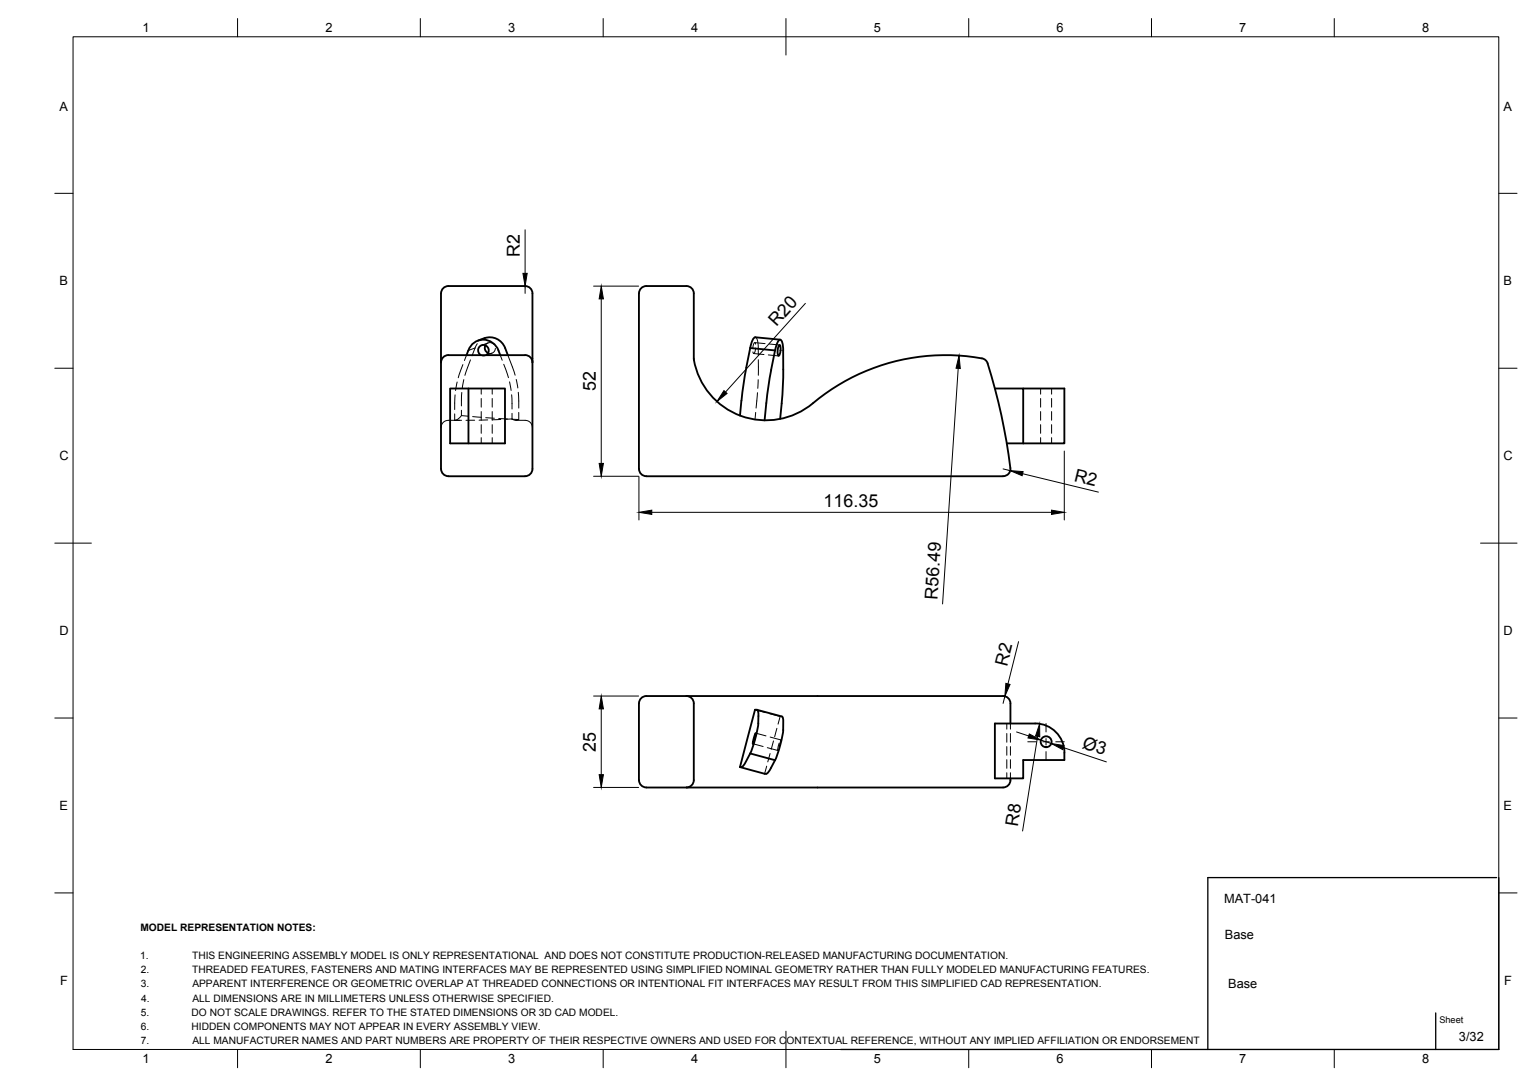
ISO-10303-21;
HEADER;
/* Generated by software containing ST-Developer
 * from STEP Tools, Inc. (www.steptools.com) 
 */

FILE_DESCRIPTION(
/* description */ ('STEP AP214'),
/* implementation_level */ '2;1');

FILE_NAME(
/* name */ 'Base.step',
/* time_stamp */ '2026-11-14T21:57:47-08:00',
/* author */ (''),
/* organization */ (''),
/* preprocessor_version */ 'ST-DEVELOPER v20.2',
/* originating_system */ 'Autodesk Translation Framework v15.17.0.0',
/* authorisation */ '');

FILE_SCHEMA (('AUTOMOTIVE_DESIGN { 1 0 10303 214 3 1 1 }'));
ENDSEC;

DATA;
#10=MECHANICAL_DESIGN_GEOMETRIC_PRESENTATION_REPRESENTATION('',(#248),#13199);
#212=SHAPE_REPRESENTATION_RELATIONSHIP('SRR','None',#13279,#230);
#230=ADVANCED_BREP_SHAPE_REPRESENTATION('',(#266),#13175);
#248=STYLED_ITEM('',(#13408),#266);
#266=MANIFOLD_SOLID_BREP('Body1',#6843);
#284=FACE_BOUND('',#2199,.T.);
#285=FACE_BOUND('',#2202,.T.);
#286=FACE_BOUND('',#2204,.T.);
#287=FACE_BOUND('',#2207,.T.);
#288=FACE_BOUND('',#2215,.T.);
#289=FACE_BOUND('',#2217,.T.);
#383=ELLIPSE('',#7086,20.7055236081625,19.9999999999245);
#384=ELLIPSE('',#7091,77.2740661068614,20.0000000018389);
#385=ELLIPSE('',#7093,20.7055236081649,19.9999999999297);
#386=ELLIPSE('',#7096,77.2740661044132,20.0000000006464);
#397=PLANE('',#7085);
#398=PLANE('',#7087);
#399=PLANE('',#7092);
#400=PLANE('',#7094);
#401=PLANE('',#7104);
#402=PLANE('',#7106);
#403=PLANE('',#7107);
#404=PLANE('',#7108);
#405=PLANE('',#7109);
#406=PLANE('',#7110);
#407=PLANE('',#7114);
#408=PLANE('',#7118);
#409=PLANE('',#7120);
#410=PLANE('',#7122);
#411=PLANE('',#7123);
#412=PLANE('',#7125);
#413=PLANE('',#7126);
#414=PLANE('',#7188);
#415=PLANE('',#7189);
#610=LINE('',#9916,#1128);
#611=LINE('',#9922,#1129);
#612=LINE('',#9928,#1130);
#613=LINE('',#9930,#1131);
#614=LINE('',#9934,#1132);
#615=LINE('',#9936,#1133);
#616=LINE('',#9938,#1134);
#617=LINE('',#9943,#1135);
#618=LINE('',#9947,#1136);
#619=LINE('',#9951,#1137);
#620=LINE('',#9957,#1138);
#621=LINE('',#9958,#1139);
#622=LINE('',#9963,#1140);
#623=LINE('',#9969,#1141);
#624=LINE('',#9975,#1142);
#625=LINE('',#9978,#1143);
#626=LINE('',#9981,#1144);
#627=LINE('',#9985,#1145);
#628=LINE('',#9990,#1146);
#629=LINE('',#9992,#1147);
#630=LINE('',#9994,#1148);
#631=LINE('',#9995,#1149);
#632=LINE('',#9997,#1150);
#633=LINE('',#10001,#1151);
#634=LINE('',#10003,#1152);
#635=LINE('',#10005,#1153);
#636=LINE('',#10006,#1154);
#637=LINE('',#10010,#1155);
#638=LINE('',#10012,#1156);
#639=LINE('',#10014,#1157);
#640=LINE('',#10015,#1158);
#641=LINE('',#10019,#1159);
#642=LINE('',#10021,#1160);
#643=LINE('',#10023,#1161);
#644=LINE('',#10024,#1162);
#645=LINE('',#10028,#1163);
#646=LINE('',#10030,#1164);
#647=LINE('',#10031,#1165);
#648=LINE('',#10032,#1166);
#649=LINE('',#10041,#1167);
#650=LINE('',#10043,#1168);
#651=LINE('',#10045,#1169);
#652=LINE('',#10046,#1170);
#653=LINE('',#10054,#1171);
#654=LINE('',#10056,#1172);
#655=LINE('',#10058,#1173);
#656=LINE('',#10059,#1174);
#657=LINE('',#10062,#1175);
#658=LINE('',#10065,#1176);
#659=LINE('',#10067,#1177);
#660=LINE('',#10068,#1178);
#661=LINE('',#10071,#1179);
#662=LINE('',#10074,#1180);
#663=LINE('',#10076,#1181);
#664=LINE('',#10077,#1182);
#665=LINE('',#10079,#1183);
#666=LINE('',#10081,#1184);
#667=LINE('',#10084,#1185);
#668=LINE('',#10147,#1186);
#669=LINE('',#10148,#1187);
#670=LINE('',#10150,#1188);
#671=LINE('',#10152,#1189);
#1128=VECTOR('',#7865,1.5);
#1129=VECTOR('',#7872,1.5);
#1130=VECTOR('',#7879,1000.);
#1131=VECTOR('',#7882,1000.);
#1132=VECTOR('',#7885,1000.);
#1133=VECTOR('',#7886,1000.);
#1134=VECTOR('',#7887,1000.);
#1135=VECTOR('',#7892,1000.);
#1136=VECTOR('',#7895,1000.);
#1137=VECTOR('',#7898,1000.);
#1138=VECTOR('',#7905,1000.);
#1139=VECTOR('',#7906,1000.);
#1140=VECTOR('',#7911,1000.);
#1141=VECTOR('',#7918,1000.);
#1142=VECTOR('',#7925,1000.);
#1143=VECTOR('',#7928,1000.);
#1144=VECTOR('',#7929,1000.);
#1145=VECTOR('',#7932,1000.);
#1146=VECTOR('',#7937,1000.);
#1147=VECTOR('',#7938,1000.);
#1148=VECTOR('',#7939,1000.);
#1149=VECTOR('',#7940,1000.);
#1150=VECTOR('',#7943,1000.);
#1151=VECTOR('',#7946,1000.);
#1152=VECTOR('',#7947,1000.);
#1153=VECTOR('',#7948,1000.);
#1154=VECTOR('',#7949,1000.);
#1155=VECTOR('',#7952,1000.);
#1156=VECTOR('',#7953,1000.);
#1157=VECTOR('',#7954,1000.);
#1158=VECTOR('',#7955,1000.);
#1159=VECTOR('',#7958,1000.);
#1160=VECTOR('',#7959,1000.);
#1161=VECTOR('',#7960,1000.);
#1162=VECTOR('',#7961,1000.);
#1163=VECTOR('',#7964,1000.);
#1164=VECTOR('',#7965,1000.);
#1165=VECTOR('',#7966,1000.);
#1166=VECTOR('',#7967,1000.);
#1167=VECTOR('',#7976,1000.);
#1168=VECTOR('',#7977,1000.);
#1169=VECTOR('',#7978,1000.);
#1170=VECTOR('',#7979,1000.);
#1171=VECTOR('',#7988,1000.);
#1172=VECTOR('',#7989,1000.);
#1173=VECTOR('',#7990,1000.);
#1174=VECTOR('',#7991,1000.);
#1175=VECTOR('',#7994,1000.);
#1176=VECTOR('',#7997,1000.);
#1177=VECTOR('',#7998,1000.);
#1178=VECTOR('',#7999,1000.);
#1179=VECTOR('',#8002,1000.);
#1180=VECTOR('',#8005,1000.);
#1181=VECTOR('',#8006,1000.);
#1182=VECTOR('',#8007,1000.);
#1183=VECTOR('',#8010,1000.);
#1184=VECTOR('',#8013,1000.);
#1185=VECTOR('',#8018,1000.);
#1186=VECTOR('',#8143,1000.);
#1187=VECTOR('',#8144,1000.);
#1188=VECTOR('',#8147,1000.);
#1189=VECTOR('',#8150,1000.);
#1646=CYLINDRICAL_SURFACE('',#7076,1.5);
#1647=CYLINDRICAL_SURFACE('',#7079,1.5);
#1648=CYLINDRICAL_SURFACE('',#7082,56.4897440054506);
#1649=CYLINDRICAL_SURFACE('',#7099,163.25688730188);
#1650=CYLINDRICAL_SURFACE('',#7105,20.);
#1651=CYLINDRICAL_SURFACE('',#7124,8.);
#1652=CYLINDRICAL_SURFACE('',#7127,2.);
#1653=CYLINDRICAL_SURFACE('',#7136,2.);
#1654=CYLINDRICAL_SURFACE('',#7138,2.);
#1655=CYLINDRICAL_SURFACE('',#7140,2.);
#1656=CYLINDRICAL_SURFACE('',#7141,2.);
#1657=CYLINDRICAL_SURFACE('',#7143,2.);
#1658=CYLINDRICAL_SURFACE('',#7153,2.);
#1659=CYLINDRICAL_SURFACE('',#7155,2.);
#1660=CYLINDRICAL_SURFACE('',#7157,2.);
#1661=CYLINDRICAL_SURFACE('',#7163,2.);
#1662=CYLINDRICAL_SURFACE('',#7165,2.);
#1663=CYLINDRICAL_SURFACE('',#7175,2.);
#1664=CYLINDRICAL_SURFACE('',#7177,2.);
#1665=CYLINDRICAL_SURFACE('',#7179,2.);
#1666=CYLINDRICAL_SURFACE('',#7187,4.54881469766181);
#1667=CYLINDRICAL_SURFACE('',#7190,25.);
#1668=CYLINDRICAL_SURFACE('',#7191,25.);
#1789=SPHERICAL_SURFACE('',#7072,2.);
#1790=SPHERICAL_SURFACE('',#7130,2.);
#1791=SPHERICAL_SURFACE('',#7133,2.);
#1792=SPHERICAL_SURFACE('',#7146,2.);
#1793=SPHERICAL_SURFACE('',#7148,2.);
#1794=SPHERICAL_SURFACE('',#7151,2.);
#1795=SPHERICAL_SURFACE('',#7167,2.);
#1796=SPHERICAL_SURFACE('',#7171,2.);
#1797=SPHERICAL_SURFACE('',#7173,2.);
#1798=SPHERICAL_SURFACE('',#7184,2.);
#1800=FACE_OUTER_BOUND('',#2191,.T.);
#1801=FACE_OUTER_BOUND('',#2192,.T.);
#1802=FACE_OUTER_BOUND('',#2193,.T.);
#1803=FACE_OUTER_BOUND('',#2194,.T.);
#1804=FACE_OUTER_BOUND('',#2195,.T.);
#1805=FACE_OUTER_BOUND('',#2196,.T.);
#1806=FACE_OUTER_BOUND('',#2197,.T.);
#1807=FACE_OUTER_BOUND('',#2198,.T.);
#1808=FACE_OUTER_BOUND('',#2200,.T.);
#1809=FACE_OUTER_BOUND('',#2201,.T.);
#1810=FACE_OUTER_BOUND('',#2203,.T.);
#1811=FACE_OUTER_BOUND('',#2205,.T.);
#1812=FACE_OUTER_BOUND('',#2206,.T.);
#1813=FACE_OUTER_BOUND('',#2208,.T.);
#1814=FACE_OUTER_BOUND('',#2209,.T.);
#1815=FACE_OUTER_BOUND('',#2210,.T.);
#1816=FACE_OUTER_BOUND('',#2211,.T.);
#1817=FACE_OUTER_BOUND('',#2212,.T.);
#1818=FACE_OUTER_BOUND('',#2213,.T.);
#1819=FACE_OUTER_BOUND('',#2214,.T.);
#1820=FACE_OUTER_BOUND('',#2216,.T.);
#1821=FACE_OUTER_BOUND('',#2218,.T.);
#1822=FACE_OUTER_BOUND('',#2219,.T.);
#1823=FACE_OUTER_BOUND('',#2220,.T.);
#1824=FACE_OUTER_BOUND('',#2221,.T.);
#1825=FACE_OUTER_BOUND('',#2222,.T.);
#1826=FACE_OUTER_BOUND('',#2223,.T.);
#1827=FACE_OUTER_BOUND('',#2224,.T.);
#1828=FACE_OUTER_BOUND('',#2225,.T.);
#1829=FACE_OUTER_BOUND('',#2226,.T.);
#1830=FACE_OUTER_BOUND('',#2227,.T.);
#1831=FACE_OUTER_BOUND('',#2228,.T.);
#1832=FACE_OUTER_BOUND('',#2229,.T.);
#1833=FACE_OUTER_BOUND('',#2230,.T.);
#1834=FACE_OUTER_BOUND('',#2231,.T.);
#1835=FACE_OUTER_BOUND('',#2232,.T.);
#1836=FACE_OUTER_BOUND('',#2233,.T.);
#1837=FACE_OUTER_BOUND('',#2234,.T.);
#1838=FACE_OUTER_BOUND('',#2235,.T.);
#1839=FACE_OUTER_BOUND('',#2236,.T.);
#1840=FACE_OUTER_BOUND('',#2237,.T.);
#1841=FACE_OUTER_BOUND('',#2238,.T.);
#1842=FACE_OUTER_BOUND('',#2239,.T.);
#1843=FACE_OUTER_BOUND('',#2240,.T.);
#1844=FACE_OUTER_BOUND('',#2241,.T.);
#1845=FACE_OUTER_BOUND('',#2242,.T.);
#1846=FACE_OUTER_BOUND('',#2243,.T.);
#1847=FACE_OUTER_BOUND('',#2244,.T.);
#1848=FACE_OUTER_BOUND('',#2245,.T.);
#1849=FACE_OUTER_BOUND('',#2246,.T.);
#1850=FACE_OUTER_BOUND('',#2247,.T.);
#1851=FACE_OUTER_BOUND('',#2248,.T.);
#1852=FACE_OUTER_BOUND('',#2249,.T.);
#1853=FACE_OUTER_BOUND('',#2250,.T.);
#1854=FACE_OUTER_BOUND('',#2251,.T.);
#1855=FACE_OUTER_BOUND('',#2252,.T.);
#1856=FACE_OUTER_BOUND('',#2253,.T.);
#1857=FACE_OUTER_BOUND('',#2254,.T.);
#1858=FACE_OUTER_BOUND('',#2255,.T.);
#1859=FACE_OUTER_BOUND('',#2256,.T.);
#2191=EDGE_LOOP('',(#4558,#4559,#4560,#4561));
#2192=EDGE_LOOP('',(#4562,#4563,#4564,#4565));
#2193=EDGE_LOOP('',(#4566,#4567,#4568));
#2194=EDGE_LOOP('',(#4569,#4570,#4571,#4572));
#2195=EDGE_LOOP('',(#4573,#4574,#4575,#4576));
#2196=EDGE_LOOP('',(#4577,#4578,#4579,#4580));
#2197=EDGE_LOOP('',(#4581,#4582,#4583,#4584));
#2198=EDGE_LOOP('',(#4585,#4586,#4587,#4588,#4589,#4590,#4591,#4592));
#2199=EDGE_LOOP('',(#4593));
#2200=EDGE_LOOP('',(#4594,#4595,#4596,#4597));
#2201=EDGE_LOOP('',(#4598,#4599,#4600,#4601,#4602,#4603,#4604,#4605));
#2202=EDGE_LOOP('',(#4606));
#2203=EDGE_LOOP('',(#4607,#4608,#4609,#4610));
#2204=EDGE_LOOP('',(#4611,#4612,#4613,#4614));
#2205=EDGE_LOOP('',(#4615,#4616,#4617,#4618));
#2206=EDGE_LOOP('',(#4619,#4620,#4621,#4622));
#2207=EDGE_LOOP('',(#4623,#4624,#4625,#4626));
#2208=EDGE_LOOP('',(#4627,#4628,#4629,#4630));
#2209=EDGE_LOOP('',(#4631,#4632,#4633,#4634));
#2210=EDGE_LOOP('',(#4635,#4636,#4637,#4638));
#2211=EDGE_LOOP('',(#4639,#4640,#4641,#4642));
#2212=EDGE_LOOP('',(#4643,#4644,#4645,#4646,#4647,#4648,#4649,#4650));
#2213=EDGE_LOOP('',(#4651,#4652,#4653,#4654,#4655,#4656,#4657,#4658));
#2214=EDGE_LOOP('',(#4659,#4660,#4661,#4662,#4663,#4664,#4665));
#2215=EDGE_LOOP('',(#4666));
#2216=EDGE_LOOP('',(#4667,#4668,#4669,#4670,#4671,#4672,#4673));
#2217=EDGE_LOOP('',(#4674));
#2218=EDGE_LOOP('',(#4675,#4676,#4677,#4678));
#2219=EDGE_LOOP('',(#4679,#4680,#4681,#4682));
#2220=EDGE_LOOP('',(#4683,#4684,#4685,#4686));
#2221=EDGE_LOOP('',(#4687,#4688,#4689,#4690));
#2222=EDGE_LOOP('',(#4691,#4692,#4693,#4694));
#2223=EDGE_LOOP('',(#4695,#4696,#4697,#4698));
#2224=EDGE_LOOP('',(#4699,#4700,#4701));
#2225=EDGE_LOOP('',(#4702,#4703,#4704));
#2226=EDGE_LOOP('',(#4705,#4706,#4707,#4708));
#2227=EDGE_LOOP('',(#4709,#4710,#4711,#4712));
#2228=EDGE_LOOP('',(#4713,#4714,#4715,#4716));
#2229=EDGE_LOOP('',(#4717,#4718,#4719,#4720));
#2230=EDGE_LOOP('',(#4721,#4722,#4723,#4724));
#2231=EDGE_LOOP('',(#4725,#4726,#4727));
#2232=EDGE_LOOP('',(#4728,#4729,#4730));
#2233=EDGE_LOOP('',(#4731,#4732,#4733));
#2234=EDGE_LOOP('',(#4734,#4735,#4736,#4737));
#2235=EDGE_LOOP('',(#4738,#4739,#4740,#4741));
#2236=EDGE_LOOP('',(#4742,#4743,#4744,#4745));
#2237=EDGE_LOOP('',(#4746,#4747,#4748,#4749));
#2238=EDGE_LOOP('',(#4750,#4751,#4752,#4753));
#2239=EDGE_LOOP('',(#4754,#4755,#4756,#4757));
#2240=EDGE_LOOP('',(#4758,#4759,#4760,#4761));
#2241=EDGE_LOOP('',(#4762,#4763,#4764));
#2242=EDGE_LOOP('',(#4765,#4766,#4767,#4768));
#2243=EDGE_LOOP('',(#4769,#4770,#4771));
#2244=EDGE_LOOP('',(#4772,#4773,#4774));
#2245=EDGE_LOOP('',(#4775,#4776,#4777,#4778));
#2246=EDGE_LOOP('',(#4779,#4780,#4781,#4782));
#2247=EDGE_LOOP('',(#4783,#4784,#4785,#4786));
#2248=EDGE_LOOP('',(#4787,#4788,#4789,#4790));
#2249=EDGE_LOOP('',(#4791,#4792,#4793,#4794));
#2250=EDGE_LOOP('',(#4795,#4796,#4797));
#2251=EDGE_LOOP('',(#4798,#4799,#4800,#4801));
#2252=EDGE_LOOP('',(#4802,#4803,#4804,#4805));
#2253=EDGE_LOOP('',(#4806,#4807,#4808,#4809));
#2254=EDGE_LOOP('',(#4810,#4811,#4812,#4813));
#2255=EDGE_LOOP('',(#4814,#4815,#4816,#4817));
#2256=EDGE_LOOP('',(#4818,#4819,#4820,#4821));
#2681=CIRCLE('',#7063,22.);
#2682=CIRCLE('',#7064,2.);
#2683=CIRCLE('',#7065,20.);
#2684=CIRCLE('',#7066,2.);
#2685=CIRCLE('',#7068,20.);
#2686=CIRCLE('',#7069,2.);
#2687=CIRCLE('',#7070,22.);
#2688=CIRCLE('',#7071,2.);
#2689=CIRCLE('',#7073,2.);
#2690=CIRCLE('',#7074,2.);
#2691=CIRCLE('',#7075,2.);
#2692=CIRCLE('',#7077,1.5);
#2693=CIRCLE('',#7078,1.5);
#2694=CIRCLE('',#7080,1.5);
#2695=CIRCLE('',#7081,1.5);
#2696=CIRCLE('',#7083,56.4897440054506);
#2697=CIRCLE('',#7084,56.4897440054506);
#2698=CIRCLE('',#7088,25.);
#2699=CIRCLE('',#7089,4.54881469766181);
#2700=CIRCLE('',#7090,25.);
#2701=CIRCLE('',#7095,25.);
#2702=CIRCLE('',#7097,25.);
#2703=CIRCLE('',#7098,4.54881469766181);
#2704=CIRCLE('',#7100,163.25688730188);
#2705=CIRCLE('',#7101,163.25688730188);
#2706=CIRCLE('',#7102,163.25688730188);
#2707=CIRCLE('',#7103,163.25688730188);
#2708=CIRCLE('',#7111,161.25688730188);
#2709=CIRCLE('',#7112,54.4897440054506);
#2710=CIRCLE('',#7113,4.);
#2711=CIRCLE('',#7115,4.);
#2712=CIRCLE('',#7116,54.4897440054506);
#2713=CIRCLE('',#7117,161.25688730188);
#2714=CIRCLE('',#7119,8.);
#2715=CIRCLE('',#7121,8.00000000000001);
#2716=CIRCLE('',#7128,2.);
#2717=CIRCLE('',#7129,2.);
#2718=CIRCLE('',#7131,2.);
#2719=CIRCLE('',#7132,2.);
#2720=CIRCLE('',#7134,2.);
#2721=CIRCLE('',#7135,2.);
#2722=CIRCLE('',#7137,2.);
#2723=CIRCLE('',#7139,2.);
#2724=CIRCLE('',#7142,2.);
#2725=CIRCLE('',#7144,2.);
#2726=CIRCLE('',#7145,2.);
#2727=CIRCLE('',#7147,2.);
#2728=CIRCLE('',#7149,2.);
#2729=CIRCLE('',#7150,2.);
#2730=CIRCLE('',#7152,2.);
#2731=CIRCLE('',#7154,2.);
#2732=CIRCLE('',#7156,2.);
#2733=CIRCLE('',#7158,2.);
#2734=CIRCLE('',#7160,2.);
#2735=CIRCLE('',#7162,2.00000000000001);
#2736=CIRCLE('',#7164,2.);
#2737=CIRCLE('',#7166,2.);
#2738=CIRCLE('',#7168,2.);
#2739=CIRCLE('',#7170,2.);
#2740=CIRCLE('',#7172,2.);
#2741=CIRCLE('',#7174,2.);
#2742=CIRCLE('',#7176,2.);
#2743=CIRCLE('',#7178,2.);
#2744=CIRCLE('',#7180,2.);
#2745=CIRCLE('',#7182,2.);
#2746=CIRCLE('',#7185,2.);
#3000=VERTEX_POINT('',#9888);
#3001=VERTEX_POINT('',#9889);
#3002=VERTEX_POINT('',#9891);
#3003=VERTEX_POINT('',#9893);
#3004=VERTEX_POINT('',#9897);
#3005=VERTEX_POINT('',#9898);
#3006=VERTEX_POINT('',#9900);
#3007=VERTEX_POINT('',#9902);
#3008=VERTEX_POINT('',#9906);
#3009=VERTEX_POINT('',#9907);
#3010=VERTEX_POINT('',#9909);
#3011=VERTEX_POINT('',#9913);
#3012=VERTEX_POINT('',#9915);
#3013=VERTEX_POINT('',#9919);
#3014=VERTEX_POINT('',#9921);
#3015=VERTEX_POINT('',#9925);
#3016=VERTEX_POINT('',#9927);
#3017=VERTEX_POINT('',#9932);
#3018=VERTEX_POINT('',#9933);
#3019=VERTEX_POINT('',#9935);
#3020=VERTEX_POINT('',#9937);
#3021=VERTEX_POINT('',#9941);
#3022=VERTEX_POINT('',#9942);
#3023=VERTEX_POINT('',#9944);
#3024=VERTEX_POINT('',#9946);
#3025=VERTEX_POINT('',#9948);
#3026=VERTEX_POINT('',#9950);
#3027=VERTEX_POINT('',#9955);
#3028=VERTEX_POINT('',#9956);
#3029=VERTEX_POINT('',#9961);
#3030=VERTEX_POINT('',#9962);
#3031=VERTEX_POINT('',#9966);
#3032=VERTEX_POINT('',#9968);
#3033=VERTEX_POINT('',#9972);
#3034=VERTEX_POINT('',#9973);
#3035=VERTEX_POINT('',#9976);
#3036=VERTEX_POINT('',#9979);
#3037=VERTEX_POINT('',#9980);
#3038=VERTEX_POINT('',#9982);
#3039=VERTEX_POINT('',#9984);
#3040=VERTEX_POINT('',#9988);
#3041=VERTEX_POINT('',#9989);
#3042=VERTEX_POINT('',#9991);
#3043=VERTEX_POINT('',#9993);
#3044=VERTEX_POINT('',#9999);
#3045=VERTEX_POINT('',#10000);
#3046=VERTEX_POINT('',#10002);
#3047=VERTEX_POINT('',#10004);
#3048=VERTEX_POINT('',#10008);
#3049=VERTEX_POINT('',#10009);
#3050=VERTEX_POINT('',#10011);
#3051=VERTEX_POINT('',#10013);
#3052=VERTEX_POINT('',#10017);
#3053=VERTEX_POINT('',#10018);
#3054=VERTEX_POINT('',#10020);
#3055=VERTEX_POINT('',#10022);
#3056=VERTEX_POINT('',#10026);
#3057=VERTEX_POINT('',#10027);
#3058=VERTEX_POINT('',#10029);
#3059=VERTEX_POINT('',#10034);
#3060=VERTEX_POINT('',#10035);
#3061=VERTEX_POINT('',#10038);
#3062=VERTEX_POINT('',#10040);
#3063=VERTEX_POINT('',#10042);
#3064=VERTEX_POINT('',#10044);
#3065=VERTEX_POINT('',#10048);
#3066=VERTEX_POINT('',#10050);
#3067=VERTEX_POINT('',#10053);
#3068=VERTEX_POINT('',#10055);
#3069=VERTEX_POINT('',#10057);
#3070=VERTEX_POINT('',#10061);
#3071=VERTEX_POINT('',#10063);
#3072=VERTEX_POINT('',#10066);
#3073=VERTEX_POINT('',#10070);
#3074=VERTEX_POINT('',#10072);
#3075=VERTEX_POINT('',#10075);
#3616=EDGE_CURVE('',#3000,#3001,#2681,.T.);
#3617=EDGE_CURVE('',#3002,#3000,#2682,.T.);
#3618=EDGE_CURVE('',#3003,#3002,#2683,.T.);
#3619=EDGE_CURVE('',#3003,#3001,#2684,.T.);
#3620=EDGE_CURVE('',#3004,#3005,#2685,.T.);
#3621=EDGE_CURVE('',#3006,#3004,#2686,.T.);
#3622=EDGE_CURVE('',#3007,#3006,#2687,.T.);
#3623=EDGE_CURVE('',#3005,#3007,#2688,.T.);
#3624=EDGE_CURVE('',#3008,#3009,#2689,.T.);
#3625=EDGE_CURVE('',#3008,#3010,#2690,.T.);
#3626=EDGE_CURVE('',#3009,#3010,#2691,.T.);
#3627=EDGE_CURVE('',#3011,#3011,#2692,.T.);
#3628=EDGE_CURVE('',#3011,#3012,#610,.T.);
#3629=EDGE_CURVE('',#3012,#3012,#2693,.T.);
#3630=EDGE_CURVE('',#3013,#3013,#2694,.T.);
#3631=EDGE_CURVE('',#3013,#3014,#611,.T.);
#3632=EDGE_CURVE('',#3014,#3014,#2695,.T.);
#3633=EDGE_CURVE('',#3002,#3015,#2696,.T.);
#3634=EDGE_CURVE('',#3015,#3016,#612,.T.);
#3635=EDGE_CURVE('',#3016,#3004,#2697,.T.);
#3636=EDGE_CURVE('',#3002,#3004,#613,.T.);
#3637=EDGE_CURVE('',#3017,#3018,#614,.T.);
#3638=EDGE_CURVE('',#3017,#3019,#615,.T.);
#3639=EDGE_CURVE('',#3019,#3020,#616,.T.);
#3640=EDGE_CURVE('',#3018,#3020,#383,.T.);
#3641=EDGE_CURVE('',#3021,#3022,#617,.T.);
#3642=EDGE_CURVE('',#3021,#3023,#2698,.T.);
#3643=EDGE_CURVE('',#3023,#3024,#618,.T.);
#3644=EDGE_CURVE('',#3024,#3025,#2699,.T.);
#3645=EDGE_CURVE('',#3025,#3026,#619,.T.);
#3646=EDGE_CURVE('',#3026,#3017,#2700,.T.);
#3647=EDGE_CURVE('',#3022,#3018,#384,.T.);
#3648=EDGE_CURVE('',#3027,#3028,#620,.T.);
#3649=EDGE_CURVE('',#3027,#3021,#621,.T.);
#3650=EDGE_CURVE('',#3028,#3022,#385,.T.);
#3651=EDGE_CURVE('',#3029,#3030,#622,.T.);
#3652=EDGE_CURVE('',#3029,#3027,#2701,.T.);
#3653=EDGE_CURVE('',#3020,#3028,#386,.T.);
#3654=EDGE_CURVE('',#3019,#3031,#2702,.T.);
#3655=EDGE_CURVE('',#3032,#3031,#623,.T.);
#3656=EDGE_CURVE('',#3030,#3032,#2703,.T.);
#3657=EDGE_CURVE('',#3033,#3034,#2704,.T.);
#3658=EDGE_CURVE('',#3034,#3009,#624,.T.);
#3659=EDGE_CURVE('',#3009,#3035,#2705,.T.);
#3660=EDGE_CURVE('',#3035,#3033,#625,.T.);
#3661=EDGE_CURVE('',#3036,#3037,#626,.T.);
#3662=EDGE_CURVE('',#3038,#3037,#2706,.T.);
#3663=EDGE_CURVE('',#3039,#3038,#627,.T.);
#3664=EDGE_CURVE('',#3036,#3039,#2707,.T.);
#3665=EDGE_CURVE('',#3040,#3041,#628,.T.);
#3666=EDGE_CURVE('',#3042,#3040,#629,.T.);
#3667=EDGE_CURVE('',#3042,#3043,#630,.T.);
#3668=EDGE_CURVE('',#3041,#3043,#631,.T.);
#3669=EDGE_CURVE('',#3005,#3003,#632,.T.);
#3670=EDGE_CURVE('',#3044,#3045,#633,.T.);
#3671=EDGE_CURVE('',#3045,#3046,#634,.T.);
#3672=EDGE_CURVE('',#3046,#3047,#635,.T.);
#3673=EDGE_CURVE('',#3047,#3044,#636,.T.);
#3674=EDGE_CURVE('',#3048,#3049,#637,.T.);
#3675=EDGE_CURVE('',#3049,#3050,#638,.T.);
#3676=EDGE_CURVE('',#3050,#3051,#639,.T.);
#3677=EDGE_CURVE('',#3051,#3048,#640,.T.);
#3678=EDGE_CURVE('',#3052,#3053,#641,.T.);
#3679=EDGE_CURVE('',#3053,#3054,#642,.T.);
#3680=EDGE_CURVE('',#3054,#3055,#643,.T.);
#3681=EDGE_CURVE('',#3055,#3052,#644,.T.);
#3682=EDGE_CURVE('',#3056,#3057,#645,.T.);
#3683=EDGE_CURVE('',#3057,#3058,#646,.T.);
#3684=EDGE_CURVE('',#3058,#3008,#647,.T.);
#3685=EDGE_CURVE('',#3008,#3056,#648,.T.);
#3686=EDGE_CURVE('',#3059,#3060,#2708,.T.);
#3687=EDGE_CURVE('',#3060,#3000,#2709,.T.);
#3688=EDGE_CURVE('',#3061,#3001,#2710,.T.);
#3689=EDGE_CURVE('',#3061,#3062,#649,.T.);
#3690=EDGE_CURVE('',#3062,#3063,#650,.T.);
#3691=EDGE_CURVE('',#3063,#3064,#651,.T.);
#3692=EDGE_CURVE('',#3064,#3059,#652,.T.);
#3693=EDGE_CURVE('',#3007,#3065,#2711,.T.);
#3694=EDGE_CURVE('',#3006,#3066,#2712,.T.);
#3695=EDGE_CURVE('',#3066,#3010,#2713,.T.);
#3696=EDGE_CURVE('',#3010,#3067,#653,.T.);
#3697=EDGE_CURVE('',#3067,#3068,#654,.T.);
#3698=EDGE_CURVE('',#3068,#3069,#655,.T.);
#3699=EDGE_CURVE('',#3069,#3065,#656,.T.);
#3700=EDGE_CURVE('',#3036,#3070,#657,.T.);
#3701=EDGE_CURVE('',#3070,#3071,#2714,.T.);
#3702=EDGE_CURVE('',#3071,#3043,#658,.T.);
#3703=EDGE_CURVE('',#3072,#3042,#659,.T.);
#3704=EDGE_CURVE('',#3037,#3072,#660,.T.);
#3705=EDGE_CURVE('',#3073,#3041,#661,.T.);
#3706=EDGE_CURVE('',#3073,#3074,#2715,.T.);
#3707=EDGE_CURVE('',#3039,#3074,#662,.T.);
#3708=EDGE_CURVE('',#3075,#3038,#663,.T.);
#3709=EDGE_CURVE('',#3075,#3040,#664,.T.);
#3710=EDGE_CURVE('',#3071,#3073,#665,.T.);
#3711=EDGE_CURVE('',#3074,#3070,#666,.T.);
#3712=EDGE_CURVE('',#3072,#3075,#667,.T.);
#3713=EDGE_CURVE('',#3068,#3054,#2716,.T.);
#3714=EDGE_CURVE('',#3055,#3067,#2717,.T.);
#3715=EDGE_CURVE('',#3068,#3051,#2718,.T.);
#3716=EDGE_CURVE('',#3051,#3054,#2719,.T.);
#3717=EDGE_CURVE('',#3055,#3058,#2720,.T.);
#3718=EDGE_CURVE('',#3058,#3067,#2721,.T.);
#3719=EDGE_CURVE('',#3048,#3053,#2722,.T.);
#3720=EDGE_CURVE('',#3069,#3050,#2723,.T.);
#3721=EDGE_CURVE('',#3052,#3057,#2724,.T.);
#3722=EDGE_CURVE('',#3053,#3063,#2725,.T.);
#3723=EDGE_CURVE('',#3064,#3052,#2726,.T.);
#3724=EDGE_CURVE('',#3048,#3063,#2727,.T.);
#3725=EDGE_CURVE('',#3069,#3047,#2728,.T.);
#3726=EDGE_CURVE('',#3047,#3050,#2729,.T.);
#3727=EDGE_CURVE('',#3064,#3057,#2730,.T.);
#3728=EDGE_CURVE('',#3049,#3062,#2731,.T.);
#3729=EDGE_CURVE('',#3044,#3049,#2732,.T.);
#3730=EDGE_CURVE('',#3065,#3046,#2733,.T.);
#3731=EDGE_CURVE('',#3066,#3016,#2734,.T.);
#3732=EDGE_CURVE('',#3035,#3066,#2735,.T.);
#3733=EDGE_CURVE('',#3056,#3034,#2736,.T.);
#3734=EDGE_CURVE('',#3059,#3056,#2737,.T.);
#3735=EDGE_CURVE('',#3044,#3062,#2738,.T.);
#3736=EDGE_CURVE('',#3005,#3046,#2739,.T.);
#3737=EDGE_CURVE('',#3035,#3016,#2740,.T.);
#3738=EDGE_CURVE('',#3059,#3034,#2741,.T.);
#3739=EDGE_CURVE('',#3045,#3061,#2742,.T.);
#3740=EDGE_CURVE('',#3003,#3045,#2743,.T.);
#3741=EDGE_CURVE('',#3033,#3015,#2744,.T.);
#3742=EDGE_CURVE('',#3060,#3033,#2745,.T.);
#3743=EDGE_CURVE('',#3060,#3015,#2746,.T.);
#3744=EDGE_CURVE('',#3032,#3025,#668,.T.);
#3745=EDGE_CURVE('',#3030,#3024,#669,.T.);
#3746=EDGE_CURVE('',#3031,#3026,#670,.T.);
#3747=EDGE_CURVE('',#3023,#3029,#671,.T.);
#4558=ORIENTED_EDGE('',*,*,#3616,.F.);
#4559=ORIENTED_EDGE('',*,*,#3617,.F.);
#4560=ORIENTED_EDGE('',*,*,#3618,.F.);
#4561=ORIENTED_EDGE('',*,*,#3619,.T.);
#4562=ORIENTED_EDGE('',*,*,#3620,.F.);
#4563=ORIENTED_EDGE('',*,*,#3621,.F.);
#4564=ORIENTED_EDGE('',*,*,#3622,.F.);
#4565=ORIENTED_EDGE('',*,*,#3623,.F.);
#4566=ORIENTED_EDGE('',*,*,#3624,.F.);
#4567=ORIENTED_EDGE('',*,*,#3625,.T.);
#4568=ORIENTED_EDGE('',*,*,#3626,.F.);
#4569=ORIENTED_EDGE('',*,*,#3627,.T.);
#4570=ORIENTED_EDGE('',*,*,#3628,.T.);
#4571=ORIENTED_EDGE('',*,*,#3629,.T.);
#4572=ORIENTED_EDGE('',*,*,#3628,.F.);
#4573=ORIENTED_EDGE('',*,*,#3630,.T.);
#4574=ORIENTED_EDGE('',*,*,#3631,.T.);
#4575=ORIENTED_EDGE('',*,*,#3632,.T.);
#4576=ORIENTED_EDGE('',*,*,#3631,.F.);
#4577=ORIENTED_EDGE('',*,*,#3633,.T.);
#4578=ORIENTED_EDGE('',*,*,#3634,.T.);
#4579=ORIENTED_EDGE('',*,*,#3635,.T.);
#4580=ORIENTED_EDGE('',*,*,#3636,.F.);
#4581=ORIENTED_EDGE('',*,*,#3637,.F.);
#4582=ORIENTED_EDGE('',*,*,#3638,.T.);
#4583=ORIENTED_EDGE('',*,*,#3639,.T.);
#4584=ORIENTED_EDGE('',*,*,#3640,.F.);
#4585=ORIENTED_EDGE('',*,*,#3641,.F.);
#4586=ORIENTED_EDGE('',*,*,#3642,.T.);
#4587=ORIENTED_EDGE('',*,*,#3643,.T.);
#4588=ORIENTED_EDGE('',*,*,#3644,.T.);
#4589=ORIENTED_EDGE('',*,*,#3645,.T.);
#4590=ORIENTED_EDGE('',*,*,#3646,.T.);
#4591=ORIENTED_EDGE('',*,*,#3637,.T.);
#4592=ORIENTED_EDGE('',*,*,#3647,.F.);
#4593=ORIENTED_EDGE('',*,*,#3629,.F.);
#4594=ORIENTED_EDGE('',*,*,#3648,.F.);
#4595=ORIENTED_EDGE('',*,*,#3649,.T.);
#4596=ORIENTED_EDGE('',*,*,#3641,.T.);
#4597=ORIENTED_EDGE('',*,*,#3650,.F.);
#4598=ORIENTED_EDGE('',*,*,#3651,.F.);
#4599=ORIENTED_EDGE('',*,*,#3652,.T.);
#4600=ORIENTED_EDGE('',*,*,#3648,.T.);
#4601=ORIENTED_EDGE('',*,*,#3653,.F.);
#4602=ORIENTED_EDGE('',*,*,#3639,.F.);
#4603=ORIENTED_EDGE('',*,*,#3654,.T.);
#4604=ORIENTED_EDGE('',*,*,#3655,.F.);
#4605=ORIENTED_EDGE('',*,*,#3656,.F.);
#4606=ORIENTED_EDGE('',*,*,#3627,.F.);
#4607=ORIENTED_EDGE('',*,*,#3657,.T.);
#4608=ORIENTED_EDGE('',*,*,#3658,.T.);
#4609=ORIENTED_EDGE('',*,*,#3659,.T.);
#4610=ORIENTED_EDGE('',*,*,#3660,.T.);
#4611=ORIENTED_EDGE('',*,*,#3661,.T.);
#4612=ORIENTED_EDGE('',*,*,#3662,.F.);
#4613=ORIENTED_EDGE('',*,*,#3663,.F.);
#4614=ORIENTED_EDGE('',*,*,#3664,.F.);
#4615=ORIENTED_EDGE('',*,*,#3665,.F.);
#4616=ORIENTED_EDGE('',*,*,#3666,.F.);
#4617=ORIENTED_EDGE('',*,*,#3667,.T.);
#4618=ORIENTED_EDGE('',*,*,#3668,.F.);
#4619=ORIENTED_EDGE('',*,*,#3669,.T.);
#4620=ORIENTED_EDGE('',*,*,#3618,.T.);
#4621=ORIENTED_EDGE('',*,*,#3636,.T.);
#4622=ORIENTED_EDGE('',*,*,#3620,.T.);
#4623=ORIENTED_EDGE('',*,*,#3647,.T.);
#4624=ORIENTED_EDGE('',*,*,#3640,.T.);
#4625=ORIENTED_EDGE('',*,*,#3653,.T.);
#4626=ORIENTED_EDGE('',*,*,#3650,.T.);
#4627=ORIENTED_EDGE('',*,*,#3670,.T.);
#4628=ORIENTED_EDGE('',*,*,#3671,.T.);
#4629=ORIENTED_EDGE('',*,*,#3672,.T.);
#4630=ORIENTED_EDGE('',*,*,#3673,.T.);
#4631=ORIENTED_EDGE('',*,*,#3674,.T.);
#4632=ORIENTED_EDGE('',*,*,#3675,.T.);
#4633=ORIENTED_EDGE('',*,*,#3676,.T.);
#4634=ORIENTED_EDGE('',*,*,#3677,.T.);
#4635=ORIENTED_EDGE('',*,*,#3678,.T.);
#4636=ORIENTED_EDGE('',*,*,#3679,.T.);
#4637=ORIENTED_EDGE('',*,*,#3680,.T.);
#4638=ORIENTED_EDGE('',*,*,#3681,.T.);
#4639=ORIENTED_EDGE('',*,*,#3682,.T.);
#4640=ORIENTED_EDGE('',*,*,#3683,.T.);
#4641=ORIENTED_EDGE('',*,*,#3684,.T.);
#4642=ORIENTED_EDGE('',*,*,#3685,.T.);
#4643=ORIENTED_EDGE('',*,*,#3686,.T.);
#4644=ORIENTED_EDGE('',*,*,#3687,.T.);
#4645=ORIENTED_EDGE('',*,*,#3616,.T.);
#4646=ORIENTED_EDGE('',*,*,#3688,.F.);
#4647=ORIENTED_EDGE('',*,*,#3689,.T.);
#4648=ORIENTED_EDGE('',*,*,#3690,.T.);
#4649=ORIENTED_EDGE('',*,*,#3691,.T.);
#4650=ORIENTED_EDGE('',*,*,#3692,.T.);
#4651=ORIENTED_EDGE('',*,*,#3693,.F.);
#4652=ORIENTED_EDGE('',*,*,#3622,.T.);
#4653=ORIENTED_EDGE('',*,*,#3694,.T.);
#4654=ORIENTED_EDGE('',*,*,#3695,.T.);
#4655=ORIENTED_EDGE('',*,*,#3696,.T.);
#4656=ORIENTED_EDGE('',*,*,#3697,.T.);
#4657=ORIENTED_EDGE('',*,*,#3698,.T.);
#4658=ORIENTED_EDGE('',*,*,#3699,.T.);
#4659=ORIENTED_EDGE('',*,*,#3700,.T.);
#4660=ORIENTED_EDGE('',*,*,#3701,.T.);
#4661=ORIENTED_EDGE('',*,*,#3702,.T.);
#4662=ORIENTED_EDGE('',*,*,#3667,.F.);
#4663=ORIENTED_EDGE('',*,*,#3703,.F.);
#4664=ORIENTED_EDGE('',*,*,#3704,.F.);
#4665=ORIENTED_EDGE('',*,*,#3661,.F.);
#4666=ORIENTED_EDGE('',*,*,#3630,.F.);
#4667=ORIENTED_EDGE('',*,*,#3705,.F.);
#4668=ORIENTED_EDGE('',*,*,#3706,.T.);
#4669=ORIENTED_EDGE('',*,*,#3707,.F.);
#4670=ORIENTED_EDGE('',*,*,#3663,.T.);
#4671=ORIENTED_EDGE('',*,*,#3708,.F.);
#4672=ORIENTED_EDGE('',*,*,#3709,.T.);
#4673=ORIENTED_EDGE('',*,*,#3665,.T.);
#4674=ORIENTED_EDGE('',*,*,#3632,.F.);
#4675=ORIENTED_EDGE('',*,*,#3702,.F.);
#4676=ORIENTED_EDGE('',*,*,#3710,.T.);
#4677=ORIENTED_EDGE('',*,*,#3705,.T.);
#4678=ORIENTED_EDGE('',*,*,#3668,.T.);
#4679=ORIENTED_EDGE('',*,*,#3707,.T.);
#4680=ORIENTED_EDGE('',*,*,#3711,.T.);
#4681=ORIENTED_EDGE('',*,*,#3700,.F.);
#4682=ORIENTED_EDGE('',*,*,#3664,.T.);
#4683=ORIENTED_EDGE('',*,*,#3706,.F.);
#4684=ORIENTED_EDGE('',*,*,#3710,.F.);
#4685=ORIENTED_EDGE('',*,*,#3701,.F.);
#4686=ORIENTED_EDGE('',*,*,#3711,.F.);
#4687=ORIENTED_EDGE('',*,*,#3666,.T.);
#4688=ORIENTED_EDGE('',*,*,#3709,.F.);
#4689=ORIENTED_EDGE('',*,*,#3712,.F.);
#4690=ORIENTED_EDGE('',*,*,#3703,.T.);
#4691=ORIENTED_EDGE('',*,*,#3662,.T.);
#4692=ORIENTED_EDGE('',*,*,#3704,.T.);
#4693=ORIENTED_EDGE('',*,*,#3712,.T.);
#4694=ORIENTED_EDGE('',*,*,#3708,.T.);
#4695=ORIENTED_EDGE('',*,*,#3713,.F.);
#4696=ORIENTED_EDGE('',*,*,#3697,.F.);
#4697=ORIENTED_EDGE('',*,*,#3714,.F.);
#4698=ORIENTED_EDGE('',*,*,#3680,.F.);
#4699=ORIENTED_EDGE('',*,*,#3715,.F.);
#4700=ORIENTED_EDGE('',*,*,#3713,.T.);
#4701=ORIENTED_EDGE('',*,*,#3716,.F.);
#4702=ORIENTED_EDGE('',*,*,#3717,.F.);
#4703=ORIENTED_EDGE('',*,*,#3714,.T.);
#4704=ORIENTED_EDGE('',*,*,#3718,.F.);
#4705=ORIENTED_EDGE('',*,*,#3716,.T.);
#4706=ORIENTED_EDGE('',*,*,#3679,.F.);
#4707=ORIENTED_EDGE('',*,*,#3719,.F.);
#4708=ORIENTED_EDGE('',*,*,#3677,.F.);
#4709=ORIENTED_EDGE('',*,*,#3715,.T.);
#4710=ORIENTED_EDGE('',*,*,#3676,.F.);
#4711=ORIENTED_EDGE('',*,*,#3720,.F.);
#4712=ORIENTED_EDGE('',*,*,#3698,.F.);
#4713=ORIENTED_EDGE('',*,*,#3718,.T.);
#4714=ORIENTED_EDGE('',*,*,#3696,.F.);
#4715=ORIENTED_EDGE('',*,*,#3625,.F.);
#4716=ORIENTED_EDGE('',*,*,#3684,.F.);
#4717=ORIENTED_EDGE('',*,*,#3717,.T.);
#4718=ORIENTED_EDGE('',*,*,#3683,.F.);
#4719=ORIENTED_EDGE('',*,*,#3721,.F.);
#4720=ORIENTED_EDGE('',*,*,#3681,.F.);
#4721=ORIENTED_EDGE('',*,*,#3722,.F.);
#4722=ORIENTED_EDGE('',*,*,#3678,.F.);
#4723=ORIENTED_EDGE('',*,*,#3723,.F.);
#4724=ORIENTED_EDGE('',*,*,#3691,.F.);
#4725=ORIENTED_EDGE('',*,*,#3719,.T.);
#4726=ORIENTED_EDGE('',*,*,#3722,.T.);
#4727=ORIENTED_EDGE('',*,*,#3724,.F.);
#4728=ORIENTED_EDGE('',*,*,#3725,.F.);
#4729=ORIENTED_EDGE('',*,*,#3720,.T.);
#4730=ORIENTED_EDGE('',*,*,#3726,.F.);
#4731=ORIENTED_EDGE('',*,*,#3723,.T.);
#4732=ORIENTED_EDGE('',*,*,#3721,.T.);
#4733=ORIENTED_EDGE('',*,*,#3727,.F.);
#4734=ORIENTED_EDGE('',*,*,#3724,.T.);
#4735=ORIENTED_EDGE('',*,*,#3690,.F.);
#4736=ORIENTED_EDGE('',*,*,#3728,.F.);
#4737=ORIENTED_EDGE('',*,*,#3674,.F.);
#4738=ORIENTED_EDGE('',*,*,#3726,.T.);
#4739=ORIENTED_EDGE('',*,*,#3675,.F.);
#4740=ORIENTED_EDGE('',*,*,#3729,.F.);
#4741=ORIENTED_EDGE('',*,*,#3673,.F.);
#4742=ORIENTED_EDGE('',*,*,#3725,.T.);
#4743=ORIENTED_EDGE('',*,*,#3672,.F.);
#4744=ORIENTED_EDGE('',*,*,#3730,.F.);
#4745=ORIENTED_EDGE('',*,*,#3699,.F.);
#4746=ORIENTED_EDGE('',*,*,#3621,.T.);
#4747=ORIENTED_EDGE('',*,*,#3635,.F.);
#4748=ORIENTED_EDGE('',*,*,#3731,.F.);
#4749=ORIENTED_EDGE('',*,*,#3694,.F.);
#4750=ORIENTED_EDGE('',*,*,#3626,.T.);
#4751=ORIENTED_EDGE('',*,*,#3695,.F.);
#4752=ORIENTED_EDGE('',*,*,#3732,.F.);
#4753=ORIENTED_EDGE('',*,*,#3659,.F.);
#4754=ORIENTED_EDGE('',*,*,#3624,.T.);
#4755=ORIENTED_EDGE('',*,*,#3658,.F.);
#4756=ORIENTED_EDGE('',*,*,#3733,.F.);
#4757=ORIENTED_EDGE('',*,*,#3685,.F.);
#4758=ORIENTED_EDGE('',*,*,#3727,.T.);
#4759=ORIENTED_EDGE('',*,*,#3682,.F.);
#4760=ORIENTED_EDGE('',*,*,#3734,.F.);
#4761=ORIENTED_EDGE('',*,*,#3692,.F.);
#4762=ORIENTED_EDGE('',*,*,#3729,.T.);
#4763=ORIENTED_EDGE('',*,*,#3728,.T.);
#4764=ORIENTED_EDGE('',*,*,#3735,.F.);
#4765=ORIENTED_EDGE('',*,*,#3693,.T.);
#4766=ORIENTED_EDGE('',*,*,#3730,.T.);
#4767=ORIENTED_EDGE('',*,*,#3736,.F.);
#4768=ORIENTED_EDGE('',*,*,#3623,.T.);
#4769=ORIENTED_EDGE('',*,*,#3732,.T.);
#4770=ORIENTED_EDGE('',*,*,#3731,.T.);
#4771=ORIENTED_EDGE('',*,*,#3737,.F.);
#4772=ORIENTED_EDGE('',*,*,#3734,.T.);
#4773=ORIENTED_EDGE('',*,*,#3733,.T.);
#4774=ORIENTED_EDGE('',*,*,#3738,.F.);
#4775=ORIENTED_EDGE('',*,*,#3735,.T.);
#4776=ORIENTED_EDGE('',*,*,#3689,.F.);
#4777=ORIENTED_EDGE('',*,*,#3739,.F.);
#4778=ORIENTED_EDGE('',*,*,#3670,.F.);
#4779=ORIENTED_EDGE('',*,*,#3736,.T.);
#4780=ORIENTED_EDGE('',*,*,#3671,.F.);
#4781=ORIENTED_EDGE('',*,*,#3740,.F.);
#4782=ORIENTED_EDGE('',*,*,#3669,.F.);
#4783=ORIENTED_EDGE('',*,*,#3737,.T.);
#4784=ORIENTED_EDGE('',*,*,#3634,.F.);
#4785=ORIENTED_EDGE('',*,*,#3741,.F.);
#4786=ORIENTED_EDGE('',*,*,#3660,.F.);
#4787=ORIENTED_EDGE('',*,*,#3738,.T.);
#4788=ORIENTED_EDGE('',*,*,#3657,.F.);
#4789=ORIENTED_EDGE('',*,*,#3742,.F.);
#4790=ORIENTED_EDGE('',*,*,#3686,.F.);
#4791=ORIENTED_EDGE('',*,*,#3739,.T.);
#4792=ORIENTED_EDGE('',*,*,#3688,.T.);
#4793=ORIENTED_EDGE('',*,*,#3619,.F.);
#4794=ORIENTED_EDGE('',*,*,#3740,.T.);
#4795=ORIENTED_EDGE('',*,*,#3742,.T.);
#4796=ORIENTED_EDGE('',*,*,#3741,.T.);
#4797=ORIENTED_EDGE('',*,*,#3743,.F.);
#4798=ORIENTED_EDGE('',*,*,#3743,.T.);
#4799=ORIENTED_EDGE('',*,*,#3633,.F.);
#4800=ORIENTED_EDGE('',*,*,#3617,.T.);
#4801=ORIENTED_EDGE('',*,*,#3687,.F.);
#4802=ORIENTED_EDGE('',*,*,#3656,.T.);
#4803=ORIENTED_EDGE('',*,*,#3744,.T.);
#4804=ORIENTED_EDGE('',*,*,#3644,.F.);
#4805=ORIENTED_EDGE('',*,*,#3745,.F.);
#4806=ORIENTED_EDGE('',*,*,#3655,.T.);
#4807=ORIENTED_EDGE('',*,*,#3746,.T.);
#4808=ORIENTED_EDGE('',*,*,#3645,.F.);
#4809=ORIENTED_EDGE('',*,*,#3744,.F.);
#4810=ORIENTED_EDGE('',*,*,#3643,.F.);
#4811=ORIENTED_EDGE('',*,*,#3747,.T.);
#4812=ORIENTED_EDGE('',*,*,#3651,.T.);
#4813=ORIENTED_EDGE('',*,*,#3745,.T.);
#4814=ORIENTED_EDGE('',*,*,#3652,.F.);
#4815=ORIENTED_EDGE('',*,*,#3747,.F.);
#4816=ORIENTED_EDGE('',*,*,#3642,.F.);
#4817=ORIENTED_EDGE('',*,*,#3649,.F.);
#4818=ORIENTED_EDGE('',*,*,#3654,.F.);
#4819=ORIENTED_EDGE('',*,*,#3638,.F.);
#4820=ORIENTED_EDGE('',*,*,#3646,.F.);
#4821=ORIENTED_EDGE('',*,*,#3746,.F.);
#6442=TOROIDAL_SURFACE('',#7062,22.,2.);
#6443=TOROIDAL_SURFACE('',#7067,22.,2.);
#6444=TOROIDAL_SURFACE('',#7159,54.4897440054506,2.);
#6445=TOROIDAL_SURFACE('',#7161,161.25688730188,2.);
#6446=TOROIDAL_SURFACE('',#7169,4.,2.);
#6447=TOROIDAL_SURFACE('',#7181,161.25688730188,2.);
#6448=TOROIDAL_SURFACE('',#7183,4.,2.);
#6449=TOROIDAL_SURFACE('',#7186,54.4897440054506,2.);
#6452=ADVANCED_FACE('',(#1800),#6442,.T.);
#6453=ADVANCED_FACE('',(#1801),#6443,.T.);
#6454=ADVANCED_FACE('',(#1802),#1789,.T.);
#6455=ADVANCED_FACE('',(#1803),#1646,.F.);
#6456=ADVANCED_FACE('',(#1804),#1647,.F.);
#6457=ADVANCED_FACE('',(#1805),#1648,.T.);
#6458=ADVANCED_FACE('',(#1806),#397,.T.);
#6459=ADVANCED_FACE('',(#1807,#284),#398,.T.);
#6460=ADVANCED_FACE('',(#1808),#399,.T.);
#6461=ADVANCED_FACE('',(#1809,#285),#400,.T.);
#6462=ADVANCED_FACE('',(#1810,#286),#1649,.T.);
#6463=ADVANCED_FACE('',(#1811),#401,.T.);
#6464=ADVANCED_FACE('',(#1812,#287),#1650,.F.);
#6465=ADVANCED_FACE('',(#1813),#402,.F.);
#6466=ADVANCED_FACE('',(#1814),#403,.F.);
#6467=ADVANCED_FACE('',(#1815),#404,.F.);
#6468=ADVANCED_FACE('',(#1816),#405,.F.);
#6469=ADVANCED_FACE('',(#1817),#406,.T.);
#6470=ADVANCED_FACE('',(#1818),#407,.F.);
#6471=ADVANCED_FACE('',(#1819,#288),#408,.T.);
#6472=ADVANCED_FACE('',(#1820,#289),#409,.F.);
#6473=ADVANCED_FACE('',(#1821),#410,.F.);
#6474=ADVANCED_FACE('',(#1822),#411,.F.);
#6475=ADVANCED_FACE('',(#1823),#1651,.T.);
#6476=ADVANCED_FACE('',(#1824),#412,.F.);
#6477=ADVANCED_FACE('',(#1825),#413,.T.);
#6478=ADVANCED_FACE('',(#1826),#1652,.T.);
#6479=ADVANCED_FACE('',(#1827),#1790,.T.);
#6480=ADVANCED_FACE('',(#1828),#1791,.T.);
#6481=ADVANCED_FACE('',(#1829),#1653,.T.);
#6482=ADVANCED_FACE('',(#1830),#1654,.T.);
#6483=ADVANCED_FACE('',(#1831),#1655,.T.);
#6484=ADVANCED_FACE('',(#1832),#1656,.T.);
#6485=ADVANCED_FACE('',(#1833),#1657,.T.);
#6486=ADVANCED_FACE('',(#1834),#1792,.T.);
#6487=ADVANCED_FACE('',(#1835),#1793,.T.);
#6488=ADVANCED_FACE('',(#1836),#1794,.T.);
#6489=ADVANCED_FACE('',(#1837),#1658,.T.);
#6490=ADVANCED_FACE('',(#1838),#1659,.T.);
#6491=ADVANCED_FACE('',(#1839),#1660,.T.);
#6492=ADVANCED_FACE('',(#1840),#6444,.T.);
#6493=ADVANCED_FACE('',(#1841),#6445,.T.);
#6494=ADVANCED_FACE('',(#1842),#1661,.T.);
#6495=ADVANCED_FACE('',(#1843),#1662,.T.);
#6496=ADVANCED_FACE('',(#1844),#1795,.T.);
#6497=ADVANCED_FACE('',(#1845),#6446,.T.);
#6498=ADVANCED_FACE('',(#1846),#1796,.T.);
#6499=ADVANCED_FACE('',(#1847),#1797,.T.);
#6500=ADVANCED_FACE('',(#1848),#1663,.T.);
#6501=ADVANCED_FACE('',(#1849),#1664,.F.);
#6502=ADVANCED_FACE('',(#1850),#1665,.T.);
#6503=ADVANCED_FACE('',(#1851),#6447,.T.);
#6504=ADVANCED_FACE('',(#1852),#6448,.T.);
#6505=ADVANCED_FACE('',(#1853),#1798,.T.);
#6506=ADVANCED_FACE('',(#1854),#6449,.T.);
#6507=ADVANCED_FACE('',(#1855),#1666,.T.);
#6508=ADVANCED_FACE('',(#1856),#414,.T.);
#6509=ADVANCED_FACE('',(#1857),#415,.T.);
#6510=ADVANCED_FACE('',(#1858),#1667,.T.);
#6511=ADVANCED_FACE('',(#1859),#1668,.T.);
#6843=CLOSED_SHELL('',(#6452,#6453,#6454,#6455,#6456,#6457,#6458,#6459,
#6460,#6461,#6462,#6463,#6464,#6465,#6466,#6467,#6468,#6469,#6470,#6471,
#6472,#6473,#6474,#6475,#6476,#6477,#6478,#6479,#6480,#6481,#6482,#6483,
#6484,#6485,#6486,#6487,#6488,#6489,#6490,#6491,#6492,#6493,#6494,#6495,
#6496,#6497,#6498,#6499,#6500,#6501,#6502,#6503,#6504,#6505,#6506,#6507,
#6508,#6509,#6510,#6511));
#7061=AXIS2_PLACEMENT_3D('',#9886,#7831,#7832);
#7062=AXIS2_PLACEMENT_3D('',#9887,#7833,#7834);
#7063=AXIS2_PLACEMENT_3D('',#9890,#7835,#7836);
#7064=AXIS2_PLACEMENT_3D('',#9892,#7837,#7838);
#7065=AXIS2_PLACEMENT_3D('',#9894,#7839,#7840);
#7066=AXIS2_PLACEMENT_3D('',#9895,#7841,#7842);
#7067=AXIS2_PLACEMENT_3D('',#9896,#7843,#7844);
#7068=AXIS2_PLACEMENT_3D('',#9899,#7845,#7846);
#7069=AXIS2_PLACEMENT_3D('',#9901,#7847,#7848);
#7070=AXIS2_PLACEMENT_3D('',#9903,#7849,#7850);
#7071=AXIS2_PLACEMENT_3D('',#9904,#7851,#7852);
#7072=AXIS2_PLACEMENT_3D('',#9905,#7853,#7854);
#7073=AXIS2_PLACEMENT_3D('',#9908,#7855,#7856);
#7074=AXIS2_PLACEMENT_3D('',#9910,#7857,#7858);
#7075=AXIS2_PLACEMENT_3D('',#9911,#7859,#7860);
#7076=AXIS2_PLACEMENT_3D('',#9912,#7861,#7862);
#7077=AXIS2_PLACEMENT_3D('',#9914,#7863,#7864);
#7078=AXIS2_PLACEMENT_3D('',#9917,#7866,#7867);
#7079=AXIS2_PLACEMENT_3D('',#9918,#7868,#7869);
#7080=AXIS2_PLACEMENT_3D('',#9920,#7870,#7871);
#7081=AXIS2_PLACEMENT_3D('',#9923,#7873,#7874);
#7082=AXIS2_PLACEMENT_3D('',#9924,#7875,#7876);
#7083=AXIS2_PLACEMENT_3D('',#9926,#7877,#7878);
#7084=AXIS2_PLACEMENT_3D('',#9929,#7880,#7881);
#7085=AXIS2_PLACEMENT_3D('',#9931,#7883,#7884);
#7086=AXIS2_PLACEMENT_3D('',#9939,#7888,#7889);
#7087=AXIS2_PLACEMENT_3D('',#9940,#7890,#7891);
#7088=AXIS2_PLACEMENT_3D('',#9945,#7893,#7894);
#7089=AXIS2_PLACEMENT_3D('',#9949,#7896,#7897);
#7090=AXIS2_PLACEMENT_3D('',#9952,#7899,#7900);
#7091=AXIS2_PLACEMENT_3D('',#9953,#7901,#7902);
#7092=AXIS2_PLACEMENT_3D('',#9954,#7903,#7904);
#7093=AXIS2_PLACEMENT_3D('',#9959,#7907,#7908);
#7094=AXIS2_PLACEMENT_3D('',#9960,#7909,#7910);
#7095=AXIS2_PLACEMENT_3D('',#9964,#7912,#7913);
#7096=AXIS2_PLACEMENT_3D('',#9965,#7914,#7915);
#7097=AXIS2_PLACEMENT_3D('',#9967,#7916,#7917);
#7098=AXIS2_PLACEMENT_3D('',#9970,#7919,#7920);
#7099=AXIS2_PLACEMENT_3D('',#9971,#7921,#7922);
#7100=AXIS2_PLACEMENT_3D('',#9974,#7923,#7924);
#7101=AXIS2_PLACEMENT_3D('',#9977,#7926,#7927);
#7102=AXIS2_PLACEMENT_3D('',#9983,#7930,#7931);
#7103=AXIS2_PLACEMENT_3D('',#9986,#7933,#7934);
#7104=AXIS2_PLACEMENT_3D('',#9987,#7935,#7936);
#7105=AXIS2_PLACEMENT_3D('',#9996,#7941,#7942);
#7106=AXIS2_PLACEMENT_3D('',#9998,#7944,#7945);
#7107=AXIS2_PLACEMENT_3D('',#10007,#7950,#7951);
#7108=AXIS2_PLACEMENT_3D('',#10016,#7956,#7957);
#7109=AXIS2_PLACEMENT_3D('',#10025,#7962,#7963);
#7110=AXIS2_PLACEMENT_3D('',#10033,#7968,#7969);
#7111=AXIS2_PLACEMENT_3D('',#10036,#7970,#7971);
#7112=AXIS2_PLACEMENT_3D('',#10037,#7972,#7973);
#7113=AXIS2_PLACEMENT_3D('',#10039,#7974,#7975);
#7114=AXIS2_PLACEMENT_3D('',#10047,#7980,#7981);
#7115=AXIS2_PLACEMENT_3D('',#10049,#7982,#7983);
#7116=AXIS2_PLACEMENT_3D('',#10051,#7984,#7985);
#7117=AXIS2_PLACEMENT_3D('',#10052,#7986,#7987);
#7118=AXIS2_PLACEMENT_3D('',#10060,#7992,#7993);
#7119=AXIS2_PLACEMENT_3D('',#10064,#7995,#7996);
#7120=AXIS2_PLACEMENT_3D('',#10069,#8000,#8001);
#7121=AXIS2_PLACEMENT_3D('',#10073,#8003,#8004);
#7122=AXIS2_PLACEMENT_3D('',#10078,#8008,#8009);
#7123=AXIS2_PLACEMENT_3D('',#10080,#8011,#8012);
#7124=AXIS2_PLACEMENT_3D('',#10082,#8014,#8015);
#7125=AXIS2_PLACEMENT_3D('',#10083,#8016,#8017);
#7126=AXIS2_PLACEMENT_3D('',#10085,#8019,#8020);
#7127=AXIS2_PLACEMENT_3D('',#10086,#8021,#8022);
#7128=AXIS2_PLACEMENT_3D('',#10087,#8023,#8024);
#7129=AXIS2_PLACEMENT_3D('',#10088,#8025,#8026);
#7130=AXIS2_PLACEMENT_3D('',#10089,#8027,#8028);
#7131=AXIS2_PLACEMENT_3D('',#10090,#8029,#8030);
#7132=AXIS2_PLACEMENT_3D('',#10091,#8031,#8032);
#7133=AXIS2_PLACEMENT_3D('',#10092,#8033,#8034);
#7134=AXIS2_PLACEMENT_3D('',#10093,#8035,#8036);
#7135=AXIS2_PLACEMENT_3D('',#10094,#8037,#8038);
#7136=AXIS2_PLACEMENT_3D('',#10095,#8039,#8040);
#7137=AXIS2_PLACEMENT_3D('',#10096,#8041,#8042);
#7138=AXIS2_PLACEMENT_3D('',#10097,#8043,#8044);
#7139=AXIS2_PLACEMENT_3D('',#10098,#8045,#8046);
#7140=AXIS2_PLACEMENT_3D('',#10099,#8047,#8048);
#7141=AXIS2_PLACEMENT_3D('',#10100,#8049,#8050);
#7142=AXIS2_PLACEMENT_3D('',#10101,#8051,#8052);
#7143=AXIS2_PLACEMENT_3D('',#10102,#8053,#8054);
#7144=AXIS2_PLACEMENT_3D('',#10103,#8055,#8056);
#7145=AXIS2_PLACEMENT_3D('',#10104,#8057,#8058);
#7146=AXIS2_PLACEMENT_3D('',#10105,#8059,#8060);
#7147=AXIS2_PLACEMENT_3D('',#10106,#8061,#8062);
#7148=AXIS2_PLACEMENT_3D('',#10107,#8063,#8064);
#7149=AXIS2_PLACEMENT_3D('',#10108,#8065,#8066);
#7150=AXIS2_PLACEMENT_3D('',#10109,#8067,#8068);
#7151=AXIS2_PLACEMENT_3D('',#10110,#8069,#8070);
#7152=AXIS2_PLACEMENT_3D('',#10111,#8071,#8072);
#7153=AXIS2_PLACEMENT_3D('',#10112,#8073,#8074);
#7154=AXIS2_PLACEMENT_3D('',#10113,#8075,#8076);
#7155=AXIS2_PLACEMENT_3D('',#10114,#8077,#8078);
#7156=AXIS2_PLACEMENT_3D('',#10115,#8079,#8080);
#7157=AXIS2_PLACEMENT_3D('',#10116,#8081,#8082);
#7158=AXIS2_PLACEMENT_3D('',#10117,#8083,#8084);
#7159=AXIS2_PLACEMENT_3D('',#10118,#8085,#8086);
#7160=AXIS2_PLACEMENT_3D('',#10119,#8087,#8088);
#7161=AXIS2_PLACEMENT_3D('',#10120,#8089,#8090);
#7162=AXIS2_PLACEMENT_3D('',#10121,#8091,#8092);
#7163=AXIS2_PLACEMENT_3D('',#10122,#8093,#8094);
#7164=AXIS2_PLACEMENT_3D('',#10123,#8095,#8096);
#7165=AXIS2_PLACEMENT_3D('',#10124,#8097,#8098);
#7166=AXIS2_PLACEMENT_3D('',#10125,#8099,#8100);
#7167=AXIS2_PLACEMENT_3D('',#10126,#8101,#8102);
#7168=AXIS2_PLACEMENT_3D('',#10127,#8103,#8104);
#7169=AXIS2_PLACEMENT_3D('',#10128,#8105,#8106);
#7170=AXIS2_PLACEMENT_3D('',#10129,#8107,#8108);
#7171=AXIS2_PLACEMENT_3D('',#10130,#8109,#8110);
#7172=AXIS2_PLACEMENT_3D('',#10131,#8111,#8112);
#7173=AXIS2_PLACEMENT_3D('',#10132,#8113,#8114);
#7174=AXIS2_PLACEMENT_3D('',#10133,#8115,#8116);
#7175=AXIS2_PLACEMENT_3D('',#10134,#8117,#8118);
#7176=AXIS2_PLACEMENT_3D('',#10135,#8119,#8120);
#7177=AXIS2_PLACEMENT_3D('',#10136,#8121,#8122);
#7178=AXIS2_PLACEMENT_3D('',#10137,#8123,#8124);
#7179=AXIS2_PLACEMENT_3D('',#10138,#8125,#8126);
#7180=AXIS2_PLACEMENT_3D('',#10139,#8127,#8128);
#7181=AXIS2_PLACEMENT_3D('',#10140,#8129,#8130);
#7182=AXIS2_PLACEMENT_3D('',#10141,#8131,#8132);
#7183=AXIS2_PLACEMENT_3D('',#10142,#8133,#8134);
#7184=AXIS2_PLACEMENT_3D('',#10143,#8135,#8136);
#7185=AXIS2_PLACEMENT_3D('',#10144,#8137,#8138);
#7186=AXIS2_PLACEMENT_3D('',#10145,#8139,#8140);
#7187=AXIS2_PLACEMENT_3D('',#10146,#8141,#8142);
#7188=AXIS2_PLACEMENT_3D('',#10149,#8145,#8146);
#7189=AXIS2_PLACEMENT_3D('',#10151,#8148,#8149);
#7190=AXIS2_PLACEMENT_3D('',#10153,#8151,#8152);
#7191=AXIS2_PLACEMENT_3D('',#10154,#8153,#8154);
#7831=DIRECTION('axis',(0.,0.,1.));
#7832=DIRECTION('refdir',(1.,0.,0.));
#7833=DIRECTION('center_axis',(0.,0.,1.));
#7834=DIRECTION('ref_axis',(1.,0.,0.));
#7835=DIRECTION('center_axis',(0.,0.,-1.));
#7836=DIRECTION('ref_axis',(1.,0.,0.));
#7837=DIRECTION('center_axis',(-0.641775581367837,0.76689249778569,-5.56651583653725E-16));
#7838=DIRECTION('ref_axis',(-0.76689249778569,-0.641775581367837,2.9218149482617E-31));
#7839=DIRECTION('center_axis',(0.,0.,1.));
#7840=DIRECTION('ref_axis',(1.,0.,0.));
#7841=DIRECTION('center_axis',(0.984885527325901,0.173206518537793,0.));
#7842=DIRECTION('ref_axis',(0.173206518537793,-0.984885527325901,0.));
#7843=DIRECTION('center_axis',(0.,0.,1.));
#7844=DIRECTION('ref_axis',(1.,0.,0.));
#7845=DIRECTION('center_axis',(0.,0.,-1.));
#7846=DIRECTION('ref_axis',(1.,0.,0.));
#7847=DIRECTION('center_axis',(-0.641775581367838,0.76689249778569,0.));
#7848=DIRECTION('ref_axis',(-0.76689249778569,-0.641775581367838,0.));
#7849=DIRECTION('center_axis',(0.,0.,1.));
#7850=DIRECTION('ref_axis',(1.,0.,0.));
#7851=DIRECTION('center_axis',(-0.984885527325901,-0.173206518537793,0.));
#7852=DIRECTION('ref_axis',(0.173206518537793,-0.984885527325901,0.));
#7853=DIRECTION('center_axis',(1.,0.,0.));
#7854=DIRECTION('ref_axis',(0.,1.,6.88338275267597E-15));
#7855=DIRECTION('center_axis',(0.,0.,1.));
#7856=DIRECTION('ref_axis',(-1.,6.93889390390722E-15,0.));
#7857=DIRECTION('center_axis',(0.,1.,6.93889390390722E-15));
#7858=DIRECTION('ref_axis',(0.,-6.93889390390722E-15,1.));
#7859=DIRECTION('center_axis',(-0.992279004699137,-0.124025710372042,0.));
#7860=DIRECTION('ref_axis',(-0.124025710372042,0.992279004699137,0.));
#7861=DIRECTION('center_axis',(0.0933963198450884,0.961399932042651,0.25881904510252));
#7862=DIRECTION('ref_axis',(2.98017618614267E-17,-0.259955306903251,0.965620649330179));
#7863=DIRECTION('center_axis',(-0.0933963198450884,-0.961399932042651,-0.25881904510252));
#7864=DIRECTION('ref_axis',(-3.0291317207828E-17,0.259955306903251,-0.965620649330179));
#7865=DIRECTION('',(0.0933963198450884,0.961399932042651,0.25881904510252));
#7866=DIRECTION('center_axis',(0.0933963198450884,0.961399932042651,0.25881904510252));
#7867=DIRECTION('ref_axis',(2.98017618614267E-17,-0.259955306903251,0.965620649330179));
#7868=DIRECTION('center_axis',(-1.,0.,0.));
#7869=DIRECTION('ref_axis',(0.,0.,1.));
#7870=DIRECTION('center_axis',(1.,0.,0.));
#7871=DIRECTION('ref_axis',(0.,0.,-1.));
#7872=DIRECTION('',(-1.,0.,0.));
#7873=DIRECTION('center_axis',(-1.,0.,0.));
#7874=DIRECTION('ref_axis',(0.,0.,1.));
#7875=DIRECTION('center_axis',(0.,0.,-1.));
#7876=DIRECTION('ref_axis',(-1.,0.,0.));
#7877=DIRECTION('center_axis',(0.,0.,-1.));
#7878=DIRECTION('ref_axis',(1.,0.,0.));
#7879=DIRECTION('',(0.,0.,-1.));
#7880=DIRECTION('center_axis',(0.,0.,1.));
#7881=DIRECTION('ref_axis',(1.,0.,0.));
#7882=DIRECTION('',(0.,0.,-1.));
#7883=DIRECTION('center_axis',(-0.0250254684785304,-0.257606335394166,0.965925826289068));
#7884=DIRECTION('ref_axis',(1.03108140825845E-18,-0.96622843558427,-0.257687039387652));
#7885=DIRECTION('',(0.995314449491629,-0.0966909852735815,0.));
#7886=DIRECTION('',(-0.0933963198450936,-0.96139993204265,-0.258819045102522));
#7887=DIRECTION('',(0.995314449491629,-0.0966909852735815,0.));
#7888=DIRECTION('center_axis',(0.0250254684785293,0.257606335394166,-0.965925826289068));
#7889=DIRECTION('ref_axis',(0.0933963198489319,0.961399932042277,0.258819045102523));
#7890=DIRECTION('center_axis',(0.0933963198450884,0.961399932042651,0.25881904510252));
#7891=DIRECTION('ref_axis',(1.37707821742972E-18,-0.259955306903251,0.965620649330179));
#7892=DIRECTION('',(0.995314449491629,-0.0966909852735815,0.));
#7893=DIRECTION('center_axis',(0.0933963198450884,0.961399932042651,0.25881904510252));
#7894=DIRECTION('ref_axis',(3.43206474624895E-18,-0.259955306903251,0.965620649330179));
#7895=DIRECTION('',(-0.933373647950443,-0.00593445768887964,0.358857096242532));
#7896=DIRECTION('center_axis',(0.0933963198450885,0.961399932042651,0.25881904510252));
#7897=DIRECTION('ref_axis',(-2.92726432357018E-17,-0.259955306903251,0.965620649330179));
#7898=DIRECTION('',(0.917438844473794,-0.184084480291559,0.352730592331281));
#7899=DIRECTION('center_axis',(0.0933963198450884,0.961399932042651,0.25881904510252));
#7900=DIRECTION('ref_axis',(3.43206474624895E-18,-0.259955306903251,0.965620649330179));
#7901=DIRECTION('center_axis',(-0.0933963198450819,-0.961399932042651,-0.25881904510252));
#7902=DIRECTION('ref_axis',(0.0250254684833587,0.257606335393695,-0.965925826289068));
#7903=DIRECTION('center_axis',(0.0250254684785304,0.257606335394166,-0.965925826289068));
#7904=DIRECTION('ref_axis',(-1.38210229589347E-18,0.96622843558427,0.257687039387653));
#7905=DIRECTION('',(0.995314449491629,-0.0966909852735815,0.));
#7906=DIRECTION('',(0.0933963198450826,0.961399932042651,0.258819045102522));
#7907=DIRECTION('center_axis',(-0.0250254684785248,-0.257606335394166,0.965925826289068));
#7908=DIRECTION('ref_axis',(-0.0933963198403989,-0.961399932043106,-0.258819045102522));
#7909=DIRECTION('center_axis',(-0.0933963198450884,-0.961399932042651,-0.25881904510252));
#7910=DIRECTION('ref_axis',(2.59294345608955E-18,0.259955306903251,-0.965620649330179));
#7911=DIRECTION('',(-0.933373647950443,-0.00593445768887968,0.358857096242532));
#7912=DIRECTION('center_axis',(-0.0933963198450884,-0.961399932042651,-0.25881904510252));
#7913=DIRECTION('ref_axis',(9.33705359754526E-19,0.259955306903251,-0.965620649330179));
#7914=DIRECTION('center_axis',(0.0933963198450923,0.961399932042651,0.25881904510252));
#7915=DIRECTION('ref_axis',(-0.0250254684771762,-0.257606335394296,0.965925826289068));
#7916=DIRECTION('center_axis',(-0.0933963198450884,-0.961399932042651,-0.25881904510252));
#7917=DIRECTION('ref_axis',(9.33705359754526E-19,0.259955306903251,-0.965620649330179));
#7918=DIRECTION('',(0.917438844473794,-0.184084480291559,0.352730592331281));
#7919=DIRECTION('center_axis',(0.0933963198450884,0.961399932042651,0.25881904510252));
#7920=DIRECTION('ref_axis',(2.17503870714762E-17,0.259955306903251,-0.965620649330179));
#7921=DIRECTION('center_axis',(0.,0.,-1.));
#7922=DIRECTION('ref_axis',(-1.,0.,0.));
#7923=DIRECTION('center_axis',(0.,0.,-1.));
#7924=DIRECTION('ref_axis',(1.,5.35536752134463E-15,0.));
#7925=DIRECTION('',(0.,0.,-1.));
#7926=DIRECTION('center_axis',(0.,0.,1.));
#7927=DIRECTION('ref_axis',(1.,0.,0.));
#7928=DIRECTION('',(0.,0.,1.));
#7929=DIRECTION('',(0.,0.,1.));
#7930=DIRECTION('center_axis',(0.,0.,-1.));
#7931=DIRECTION('ref_axis',(1.,0.,0.));
#7932=DIRECTION('',(0.,0.,1.));
#7933=DIRECTION('center_axis',(0.,0.,1.));
#7934=DIRECTION('ref_axis',(1.,0.,0.));
#7935=DIRECTION('center_axis',(0.,0.,1.));
#7936=DIRECTION('ref_axis',(1.,0.,0.));
#7937=DIRECTION('',(-2.7390370673318E-16,1.,0.));
#7938=DIRECTION('',(-1.,0.,0.));
#7939=DIRECTION('',(0.,1.,0.));
#7940=DIRECTION('',(1.,0.,0.));
#7941=DIRECTION('center_axis',(0.,0.,-1.));
#7942=DIRECTION('ref_axis',(0.939389765090764,-0.342851089020758,0.));
#7943=DIRECTION('',(0.,0.,1.));
#7944=DIRECTION('center_axis',(1.22464679914735E-16,-1.,0.));
#7945=DIRECTION('ref_axis',(1.,1.22464679914735E-16,0.));
#7946=DIRECTION('',(1.,1.22464679914735E-16,0.));
#7947=DIRECTION('',(0.,0.,-1.));
#7948=DIRECTION('',(-1.,-1.22464679914735E-16,0.));
#7949=DIRECTION('',(0.,0.,1.));
#7950=DIRECTION('center_axis',(1.,2.31296463463574E-16,0.));
#7951=DIRECTION('ref_axis',(-2.31296463463574E-16,1.,0.));
#7952=DIRECTION('',(-2.31296463463574E-16,1.,0.));
#7953=DIRECTION('',(0.,0.,-1.));
#7954=DIRECTION('',(2.31296463463574E-16,-1.,0.));
#7955=DIRECTION('',(0.,0.,1.));
#7956=DIRECTION('center_axis',(0.,1.,0.));
#7957=DIRECTION('ref_axis',(0.,0.,1.));
#7958=DIRECTION('',(-1.,0.,0.));
#7959=DIRECTION('',(0.,0.,-1.));
#7960=DIRECTION('',(1.,0.,0.));
#7961=DIRECTION('',(0.,0.,1.));
#7962=DIRECTION('center_axis',(-1.,6.81286914308505E-17,0.));
#7963=DIRECTION('ref_axis',(-6.81286914308505E-17,-1.,0.));
#7964=DIRECTION('',(-6.81286914308505E-17,-1.,0.));
#7965=DIRECTION('',(0.,0.,-1.));
#7966=DIRECTION('',(6.81286914308505E-17,1.,0.));
#7967=DIRECTION('',(0.,0.,1.));
#7968=DIRECTION('center_axis',(0.,0.,1.));
#7969=DIRECTION('ref_axis',(1.,0.,0.));
#7970=DIRECTION('center_axis',(0.,0.,1.));
#7971=DIRECTION('ref_axis',(1.,0.,0.));
#7972=DIRECTION('center_axis',(0.,0.,1.));
#7973=DIRECTION('ref_axis',(1.,0.,0.));
#7974=DIRECTION('center_axis',(0.,0.,1.));
#7975=DIRECTION('ref_axis',(1.,0.,0.));
#7976=DIRECTION('',(-1.,-1.22464679914735E-16,0.));
#7977=DIRECTION('',(2.31296463463574E-16,-1.,0.));
#7978=DIRECTION('',(1.,0.,0.));
#7979=DIRECTION('',(6.81286914308505E-17,1.,0.));
#7980=DIRECTION('center_axis',(0.,0.,1.));
#7981=DIRECTION('ref_axis',(1.,0.,0.));
#7982=DIRECTION('center_axis',(0.,0.,-1.));
#7983=DIRECTION('ref_axis',(1.,0.,0.));
#7984=DIRECTION('center_axis',(0.,0.,-1.));
#7985=DIRECTION('ref_axis',(1.,0.,0.));
#7986=DIRECTION('center_axis',(0.,0.,-1.));
#7987=DIRECTION('ref_axis',(1.,5.33572772289561E-15,0.));
#7988=DIRECTION('',(-6.81286914308505E-17,-1.,0.));
#7989=DIRECTION('',(-1.,0.,0.));
#7990=DIRECTION('',(-2.31296463463574E-16,1.,0.));
#7991=DIRECTION('',(1.,1.22464679914735E-16,0.));
#7992=DIRECTION('center_axis',(1.,0.,0.));
#7993=DIRECTION('ref_axis',(0.,0.,-1.));
#7994=DIRECTION('',(0.,1.,0.));
#7995=DIRECTION('center_axis',(1.,0.,0.));
#7996=DIRECTION('ref_axis',(0.,0.,-1.));
#7997=DIRECTION('',(0.,0.,1.));
#7998=DIRECTION('',(0.,0.,-1.));
#7999=DIRECTION('',(0.,1.,0.));
#8000=DIRECTION('center_axis',(1.,2.7390370673318E-16,0.));
#8001=DIRECTION('ref_axis',(-2.7390370673318E-16,1.,0.));
#8002=DIRECTION('',(0.,0.,1.));
#8003=DIRECTION('center_axis',(-1.,-2.7390370673318E-16,0.));
#8004=DIRECTION('ref_axis',(-2.7390370673318E-16,1.,0.));
#8005=DIRECTION('',(-2.7390370673318E-16,1.,0.));
#8006=DIRECTION('',(-4.47852670343415E-16,-1.,0.));
#8007=DIRECTION('',(0.,0.,-1.));
#8008=DIRECTION('center_axis',(0.,-1.,0.));
#8009=DIRECTION('ref_axis',(0.,0.,-1.));
#8010=DIRECTION('',(-1.,0.,0.));
#8011=DIRECTION('center_axis',(0.,0.,1.));
#8012=DIRECTION('ref_axis',(1.,0.,0.));
#8013=DIRECTION('',(1.,0.,0.));
#8014=DIRECTION('center_axis',(1.,0.,0.));
#8015=DIRECTION('ref_axis',(0.,0.,-1.));
#8016=DIRECTION('center_axis',(0.,-1.,0.));
#8017=DIRECTION('ref_axis',(0.,0.,-1.));
#8018=DIRECTION('',(-1.,0.,0.));
#8019=DIRECTION('center_axis',(0.,0.,1.));
#8020=DIRECTION('ref_axis',(1.,0.,0.));
#8021=DIRECTION('center_axis',(1.,0.,0.));
#8022=DIRECTION('ref_axis',(0.,0.,-1.));
#8023=DIRECTION('center_axis',(-1.,0.,0.));
#8024=DIRECTION('ref_axis',(0.,0.,1.));
#8025=DIRECTION('center_axis',(1.,0.,0.));
#8026=DIRECTION('ref_axis',(0.,0.,-1.));
#8027=DIRECTION('center_axis',(1.,0.,-1.11022302462516E-16));
#8028=DIRECTION('ref_axis',(0.,-8.88178419700125E-16,-1.));
#8029=DIRECTION('center_axis',(0.,1.,0.));
#8030=DIRECTION('ref_axis',(-1.73472347597681E-15,0.,-1.));
#8031=DIRECTION('center_axis',(0.,0.,1.));
#8032=DIRECTION('ref_axis',(-1.,0.,0.));
#8033=DIRECTION('center_axis',(0.,1.,0.));
#8034=DIRECTION('ref_axis',(-1.,0.,0.));
#8035=DIRECTION('center_axis',(0.,0.,1.));
#8036=DIRECTION('ref_axis',(-1.,0.,0.));
#8037=DIRECTION('center_axis',(-1.73472347597681E-15,1.,0.));
#8038=DIRECTION('ref_axis',(1.,1.73472347597681E-15,0.));
#8039=DIRECTION('center_axis',(0.,0.,-1.));
#8040=DIRECTION('ref_axis',(-1.,0.,0.));
#8041=DIRECTION('center_axis',(0.,0.,1.));
#8042=DIRECTION('ref_axis',(1.,0.,0.));
#8043=DIRECTION('center_axis',(2.31296463463574E-16,-1.,0.));
#8044=DIRECTION('ref_axis',(1.,2.31296463463574E-16,0.));
#8045=DIRECTION('center_axis',(-2.16840434497101E-16,1.,0.));
#8046=DIRECTION('ref_axis',(-1.,-2.16840434497101E-16,0.));
#8047=DIRECTION('center_axis',(6.81286914308505E-17,1.,0.));
#8048=DIRECTION('ref_axis',(-1.,6.81286914308505E-17,0.));
#8049=DIRECTION('center_axis',(0.,0.,-1.));
#8050=DIRECTION('ref_axis',(-1.,0.,0.));
#8051=DIRECTION('center_axis',(0.,0.,1.));
#8052=DIRECTION('ref_axis',(1.,0.,0.));
#8053=DIRECTION('center_axis',(-1.,0.,0.));
#8054=DIRECTION('ref_axis',(0.,0.,1.));
#8055=DIRECTION('center_axis',(-1.,0.,-1.73472347597681E-15));
#8056=DIRECTION('ref_axis',(-1.73472347597681E-15,0.,1.));
#8057=DIRECTION('center_axis',(1.,0.,0.));
#8058=DIRECTION('ref_axis',(0.,0.,-1.));
#8059=DIRECTION('center_axis',(1.,0.,0.));
#8060=DIRECTION('ref_axis',(0.,0.,-1.));
#8061=DIRECTION('center_axis',(-1.73472347597681E-15,1.,0.));
#8062=DIRECTION('ref_axis',(1.,1.73472347597681E-15,0.));
#8063=DIRECTION('center_axis',(0.,1.,0.));
#8064=DIRECTION('ref_axis',(1.77635683940025E-15,0.,1.));
#8065=DIRECTION('center_axis',(1.,0.,0.));
#8066=DIRECTION('ref_axis',(0.,0.,1.));
#8067=DIRECTION('center_axis',(0.,0.,1.));
#8068=DIRECTION('ref_axis',(-1.,0.,0.));
#8069=DIRECTION('center_axis',(1.,0.,0.));
#8070=DIRECTION('ref_axis',(0.,0.,-1.));
#8071=DIRECTION('center_axis',(0.,1.,0.));
#8072=DIRECTION('ref_axis',(0.,0.,-1.));
#8073=DIRECTION('center_axis',(-2.31296463463574E-16,1.,0.));
#8074=DIRECTION('ref_axis',(-1.,-2.31296463463574E-16,0.));
#8075=DIRECTION('center_axis',(-2.16840434497101E-16,1.,6.50521303491302E-16));
#8076=DIRECTION('ref_axis',(-6.41463530422129E-47,-6.50521303491302E-16,
1.));
#8077=DIRECTION('center_axis',(0.,0.,-1.));
#8078=DIRECTION('ref_axis',(-1.,0.,0.));
#8079=DIRECTION('center_axis',(0.,0.,1.));
#8080=DIRECTION('ref_axis',(1.,0.,0.));
#8081=DIRECTION('center_axis',(-1.,-1.22464679914735E-16,0.));
#8082=DIRECTION('ref_axis',(1.22464679914735E-16,-1.,0.));
#8083=DIRECTION('center_axis',(1.,1.21972744404619E-16,0.));
#8084=DIRECTION('ref_axis',(-1.21972744404619E-16,1.,0.));
#8085=DIRECTION('center_axis',(0.,0.,1.));
#8086=DIRECTION('ref_axis',(-0.966517253196389,-0.25660163536834,0.));
#8087=DIRECTION('center_axis',(0.176867050811513,0.984234751640704,0.));
#8088=DIRECTION('ref_axis',(-0.984234751640704,0.176867050811512,0.));
#8089=DIRECTION('center_axis',(0.,0.,1.));
#8090=DIRECTION('ref_axis',(1.,0.,0.));
#8091=DIRECTION('center_axis',(-0.954169336796974,-0.299267232948117,8.79335597693182E-15));
#8092=DIRECTION('ref_axis',(0.299267232948117,-0.954169336796974,-6.57835715770868E-30));
#8093=DIRECTION('center_axis',(0.,0.,-1.));
#8094=DIRECTION('ref_axis',(-1.,0.,0.));
#8095=DIRECTION('center_axis',(0.,0.,1.));
#8096=DIRECTION('ref_axis',(1.,0.,0.));
#8097=DIRECTION('center_axis',(-6.81286914308505E-17,-1.,0.));
#8098=DIRECTION('ref_axis',(1.,-6.81286914308505E-17,0.));
#8099=DIRECTION('center_axis',(6.93889390390722E-15,1.,0.));
#8100=DIRECTION('ref_axis',(-1.,6.93889390390722E-15,0.));
#8101=DIRECTION('center_axis',(0.,0.,1.));
#8102=DIRECTION('ref_axis',(0.,-1.,0.));
#8103=DIRECTION('center_axis',(1.,-1.73472347597681E-15,0.));
#8104=DIRECTION('ref_axis',(-1.73472347597681E-15,-1.,0.));
#8105=DIRECTION('center_axis',(0.,0.,1.));
#8106=DIRECTION('ref_axis',(1.,0.,0.));
#8107=DIRECTION('center_axis',(0.,0.,-1.));
#8108=DIRECTION('ref_axis',(1.,0.,0.));
#8109=DIRECTION('center_axis',(-1.11022302462516E-16,1.,0.));
#8110=DIRECTION('ref_axis',(-1.,0.,8.88178419700125E-16));
#8111=DIRECTION('center_axis',(0.,0.,1.));
#8112=DIRECTION('ref_axis',(-1.,0.,0.));
#8113=DIRECTION('center_axis',(1.,0.,0.));
#8114=DIRECTION('ref_axis',(0.,-1.,7.105427357601E-15));
#8115=DIRECTION('center_axis',(-0.992279004699137,-0.124025710372042,0.));
#8116=DIRECTION('ref_axis',(-0.124025710372042,0.992279004699137,0.));
#8117=DIRECTION('center_axis',(1.,1.22464679914735E-16,0.));
#8118=DIRECTION('ref_axis',(-1.22464679914735E-16,1.,0.));
#8119=DIRECTION('center_axis',(1.,1.21972744404619E-16,7.93458686805043E-32));
#8120=DIRECTION('ref_axis',(-1.21972744404619E-16,1.,1.69964635189105E-63));
#8121=DIRECTION('center_axis',(0.,0.,-1.));
#8122=DIRECTION('ref_axis',(-1.,0.,0.));
#8123=DIRECTION('center_axis',(0.,0.,-1.));
#8124=DIRECTION('ref_axis',(1.,0.,0.));
#8125=DIRECTION('center_axis',(0.,0.,-1.));
#8126=DIRECTION('ref_axis',(-1.,0.,0.));
#8127=DIRECTION('center_axis',(0.,0.,1.));
#8128=DIRECTION('ref_axis',(1.,0.,0.));
#8129=DIRECTION('center_axis',(0.,0.,1.));
#8130=DIRECTION('ref_axis',(1.,0.,0.));
#8131=DIRECTION('center_axis',(-0.954169336796977,-0.299267232948109,0.));
#8132=DIRECTION('ref_axis',(0.299267232948109,-0.954169336796977,0.));
#8133=DIRECTION('center_axis',(0.,0.,1.));
#8134=DIRECTION('ref_axis',(1.,0.,0.));
#8135=DIRECTION('center_axis',(1.11022302462516E-16,1.,0.));
#8136=DIRECTION('ref_axis',(1.,0.,0.));
#8137=DIRECTION('center_axis',(-0.176867050811505,-0.984234751640705,-7.65406697331636E-15));
#8138=DIRECTION('ref_axis',(-0.984234751640705,0.176867050811505,4.00542835088251E-31));
#8139=DIRECTION('center_axis',(0.,0.,1.));
#8140=DIRECTION('ref_axis',(-0.966517253196389,-0.25660163536834,0.));
#8141=DIRECTION('center_axis',(0.0933963198450884,0.961399932042651,0.25881904510252));
#8142=DIRECTION('ref_axis',(2.68671235148266E-18,-0.259955306903251,0.965620649330179));
#8143=DIRECTION('',(0.0933963198450884,0.961399932042651,0.25881904510252));
#8144=DIRECTION('',(0.0933963198450884,0.961399932042651,0.25881904510252));
#8145=DIRECTION('center_axis',(-0.386759736903912,-0.204506906446147,0.899218455730221));
#8146=DIRECTION('ref_axis',(0.918633667079783,1.12376124846612E-18,0.395110346242099));
#8147=DIRECTION('',(0.0933963198450936,0.96139993204265,0.258819045102522));
#8148=DIRECTION('center_axis',(-0.346541138612831,0.275090808425737,-0.896791105201539));
#8149=DIRECTION('ref_axis',(-0.932779367662293,-3.90319787005602E-18,0.360447848188239));
#8150=DIRECTION('',(-0.0933963198450826,-0.961399932042651,-0.258819045102522));
#8151=DIRECTION('center_axis',(0.0933963198450826,0.961399932042651,0.258819045102522));
#8152=DIRECTION('ref_axis',(-0.163713918954279,0.271246303466574,-0.948484683901828));
#8153=DIRECTION('center_axis',(0.0933963198450936,0.96139993204265,0.258819045102522));
#8154=DIRECTION('ref_axis',(4.28128594136413E-18,-0.259955306903254,0.965620649330178));
#9886=CARTESIAN_POINT('',(0.,0.,0.));
#9887=CARTESIAN_POINT('Origin',(-3.28761363381793,19.7279394918662,23.));
#9888=CARTESIAN_POINT('',(13.5840213174672,33.8470022819586,25.));
#9889=CARTESIAN_POINT('',(0.522929774013513,-1.9395421093036,25.));
#9890=CARTESIAN_POINT('Origin',(-3.28761363381793,19.7279394918662,25.));
#9891=CARTESIAN_POINT('',(12.0502363218959,32.563451119223,23.));
#9892=CARTESIAN_POINT('Origin',(13.5840213174673,33.8470022819586,23.));
#9893=CARTESIAN_POINT('',(0.176516736937927,0.0302289453482035,23.));
#9894=CARTESIAN_POINT('Origin',(-3.28761363381793,19.7279394918662,23.));
#9895=CARTESIAN_POINT('Origin',(0.522929774013513,-1.9395421093036,23.));
#9896=CARTESIAN_POINT('Origin',(-3.28761363381793,19.7279394918662,2.));
#9897=CARTESIAN_POINT('',(12.0502363218959,32.563451119223,2.));
#9898=CARTESIAN_POINT('',(0.176516736937927,0.0302289453482035,2.));
#9899=CARTESIAN_POINT('Origin',(-3.28761363381793,19.7279394918662,2.));
#9900=CARTESIAN_POINT('',(13.5840213174673,33.8470022819586,0.));
#9901=CARTESIAN_POINT('Origin',(13.5840213174672,33.8470022819586,2.));
#9902=CARTESIAN_POINT('',(0.522929774013513,-1.9395421093036,0.));
#9903=CARTESIAN_POINT('Origin',(-3.28761363381793,19.7279394918662,0.));
#9904=CARTESIAN_POINT('Origin',(0.522929774013513,-1.9395421093036,2.));
#9905=CARTESIAN_POINT('Origin',(30.,84.6000761633705,2.));
#9906=CARTESIAN_POINT('',(32.,84.6000761633705,2.));
#9907=CARTESIAN_POINT('',(29.7519485792559,86.5846341727688,2.));
#9908=CARTESIAN_POINT('Origin',(30.,84.6000761633705,2.));
#9909=CARTESIAN_POINT('',(30.,84.6000761633705,0.));
#9910=CARTESIAN_POINT('Origin',(30.,84.6000761633705,2.));
#9911=CARTESIAN_POINT('Origin',(30.,84.6000761633705,2.));
#9912=CARTESIAN_POINT('Origin',(-3.32467333292967,13.7193061680048,10.8273365655636));
#9913=CARTESIAN_POINT('',(-3.05145636383197,16.9216708811215,10.136042009416));
#9914=CARTESIAN_POINT('Origin',(-3.05145636383197,16.5317379207667,11.5844729834113));
#9915=CARTESIAN_POINT('',(-2.39071013447879,23.7232384487861,11.9670960425935));
#9916=CARTESIAN_POINT('',(-3.32467333292967,14.1092391283596,9.37890559156828));
#9917=CARTESIAN_POINT('Origin',(-2.39071013447879,23.3333054884313,13.4155270165888));
#9918=CARTESIAN_POINT('Origin',(26.0000000000001,96.3501340213216,12.5));
#9919=CARTESIAN_POINT('',(23.,96.3501340213216,11.));
#9920=CARTESIAN_POINT('Origin',(23.,96.3501340213216,12.5));
#9921=CARTESIAN_POINT('',(8.00000000000006,96.3501340213216,11.));
#9922=CARTESIAN_POINT('',(26.0000000000001,96.3501340213216,11.));
#9923=CARTESIAN_POINT('Origin',(8.00000000000006,96.3501340213216,12.5));
#9924=CARTESIAN_POINT('Origin',(55.3717972015101,68.8171894196414,25.));
#9925=CARTESIAN_POINT('',(-0.227371959941596,78.8083638429823,23.));
#9926=CARTESIAN_POINT('Origin',(55.3717972015101,68.8171894196414,23.));
#9927=CARTESIAN_POINT('',(-0.227371959941596,78.8083638429823,2.));
#9928=CARTESIAN_POINT('',(-0.227371959941595,78.8083638429823,25.));
#9929=CARTESIAN_POINT('Origin',(55.3717972015101,68.8171894196414,2.));
#9930=CARTESIAN_POINT('',(12.0502363218959,32.563451119223,25.));
#9931=CARTESIAN_POINT('Origin',(-7.93301877845108,21.7616127890893,21.2536537832198));
#9932=CARTESIAN_POINT('',(11.9915524290357,19.8260170362199,21.2536537832198));
#9933=CARTESIAN_POINT('',(16.7091421738371,19.3677212677073,21.2536537832198));
#9934=CARTESIAN_POINT('',(-7.93301877845108,21.7616127890893,21.2536537832198));
#9935=CARTESIAN_POINT('',(11.3308061996825,13.0244494685553,19.4225997500424));
#9936=CARTESIAN_POINT('',(11.9915524290357,19.8260170362198,21.2536537832198));
#9937=CARTESIAN_POINT('',(15.409807546716,12.6281901161683,19.4225997500424));
#9938=CARTESIAN_POINT('',(-8.59376500780425,14.9600452214247,19.4225997500424));
#9939=CARTESIAN_POINT('Origin',(-3.28761363374331,19.7279394918536,20.831640338319));
#9940=CARTESIAN_POINT('Origin',(-7.52687414707159,25.9423708923569,5.57740024995768));
#9941=CARTESIAN_POINT('',(12.0795247373973,24.0376843616083,5.57740024995768));
#9942=CARTESIAN_POINT('',(16.3290636231184,23.6248579407434,5.57740024995768));
#9943=CARTESIAN_POINT('',(-7.52687414707159,25.9423708923569,5.57740024995768));
#9944=CARTESIAN_POINT('',(2.79035956011326,24.4747961873976,7.30576827714592));
#9945=CARTESIAN_POINT('Origin',(11.453888025434,17.5975259767542,29.7255459071844));
#9946=CARTESIAN_POINT('',(-2.39071013447879,24.4418545686223,9.2977504057545));
#9947=CARTESIAN_POINT('',(2.67091952913043,24.4740367789744,7.3516897607744));
#9948=CARTESIAN_POINT('',(-2.39071013447879,22.2247564082402,17.533303627423));
#9949=CARTESIAN_POINT('Origin',(-0.814358709812287,23.1905174560636,13.3770869658276));
#9950=CARTESIAN_POINT('',(2.94819571840111,21.1535027599203,19.5859695192486));
#9951=CARTESIAN_POINT('',(-2.29893826609133,22.206342345222,17.5685874457294));
#9952=CARTESIAN_POINT('Origin',(12.6171891409989,26.266175421074,-2.89449187400689));
#9953=CARTESIAN_POINT('Origin',(-3.28761363568232,19.7279394916906,27.1315428110125));
#9954=CARTESIAN_POINT('Origin',(-7.52687414707159,25.9423708923569,5.57740024995768));
#9955=CARTESIAN_POINT('',(11.4187785080441,17.2361167939437,3.74634621678022));
#9956=CARTESIAN_POINT('',(16.4884781618741,16.7436148968595,3.74634621678022));
#9957=CARTESIAN_POINT('',(-8.18762037642477,19.1408033246923,3.74634621678022));
#9958=CARTESIAN_POINT('',(12.0795247373973,24.0376843616084,5.57740024995771));
#9959=CARTESIAN_POINT('Origin',(-3.28761363374728,19.7279394918659,4.02988243998975));
#9960=CARTESIAN_POINT('Origin',(-8.18762037642477,19.1408033246923,3.74634621678022));
#9961=CARTESIAN_POINT('',(2.12961333076012,17.673228619733,5.47471424396846));
#9962=CARTESIAN_POINT('',(-3.05145636383197,17.6402870009577,7.46669637257706));
#9963=CARTESIAN_POINT('',(2.01017329977726,17.6724692113098,5.52063572759696));
#9964=CARTESIAN_POINT('Origin',(10.7931417960809,10.7959584090896,27.8944918740069));
#9965=CARTESIAN_POINT('Origin',(-3.28761363445173,19.7279394920272,-0.202803923569845));
#9966=CARTESIAN_POINT('',(2.2874494890479,14.3519351922557,17.7549154860712));
#9967=CARTESIAN_POINT('Origin',(11.9564429116457,19.4646078534094,-4.72554590718435));
#9968=CARTESIAN_POINT('',(-3.05145636383196,15.4231888405756,15.7022495942456));
#9969=CARTESIAN_POINT('',(-2.95968449544451,15.4047747775574,15.737533412552));
#9970=CARTESIAN_POINT('Origin',(-1.47510493916546,16.388949888399,11.5460329326502));
#9971=CARTESIAN_POINT('Origin',(50.,-75.4117474694202,25.));
#9972=CARTESIAN_POINT('',(1.14256307744359,80.3629684149532,23.));
#9973=CARTESIAN_POINT('',(29.7519485792559,86.5846341727688,23.));
#9974=CARTESIAN_POINT('Origin',(50.,-75.4117474694202,23.));
#9975=CARTESIAN_POINT('',(29.7519485792559,86.5846341727688,25.));
#9976=CARTESIAN_POINT('',(1.14256307744359,80.3629684149532,2.));
#9977=CARTESIAN_POINT('Origin',(50.,-75.4117474694202,2.));
#9978=CARTESIAN_POINT('',(1.14256307744358,80.3629684149533,25.));
#9979=CARTESIAN_POINT('',(23.,85.5969828885913,7.5));
#9980=CARTESIAN_POINT('',(23.,85.5969828885913,22.5));
#9981=CARTESIAN_POINT('',(23.,85.5969828885913,25.));
#9982=CARTESIAN_POINT('',(8.00000000000003,82.3501340213215,22.5));
#9983=CARTESIAN_POINT('Origin',(50.,-75.4117474694202,22.5));
#9984=CARTESIAN_POINT('',(8.00000000000004,82.3501340213216,7.5));
#9985=CARTESIAN_POINT('',(8.00000000000004,82.3501340213216,7.5));
#9986=CARTESIAN_POINT('Origin',(50.,-75.4117474694202,7.5));
#9987=CARTESIAN_POINT('Origin',(0.,0.,17.5));
#9988=CARTESIAN_POINT('',(8.00000000000003,90.0969828885913,17.5));
#9989=CARTESIAN_POINT('',(8.00000000000003,101.350134021322,17.5));
#9990=CARTESIAN_POINT('',(8.00000000000006,2.19122965386546E-15,17.5));
#9991=CARTESIAN_POINT('',(23.,90.0969828885913,17.5));
#9992=CARTESIAN_POINT('',(8.00000000000004,90.0969828885913,17.5));
#9993=CARTESIAN_POINT('',(23.,101.350134021322,17.5));
#9994=CARTESIAN_POINT('',(23.,0.,17.5));
#9995=CARTESIAN_POINT('',(0.,101.350134021322,17.5));
#9996=CARTESIAN_POINT('Origin',(-3.28761363381793,19.7279394918662,25.));
#9997=CARTESIAN_POINT('',(0.176516736937928,0.0302289453482027,25.));
#9998=CARTESIAN_POINT('Origin',(0.,0.,25.));
#9999=CARTESIAN_POINT('',(-18.,-2.20436423846524E-15,23.));
#10000=CARTESIAN_POINT('',(-0.169896300137657,-2.0806296015056E-17,23.));
#10001=CARTESIAN_POINT('',(1.88751509164731E-16,2.3115393153282E-32,23.));
#10002=CARTESIAN_POINT('',(-0.169896300137657,-2.0806296015056E-17,2.));
#10003=CARTESIAN_POINT('',(-0.169896300137657,-2.0806296015056E-17,0.));
#10004=CARTESIAN_POINT('',(-18.,-2.20436423846524E-15,2.));
#10005=CARTESIAN_POINT('',(0.,0.,2.));
#10006=CARTESIAN_POINT('',(-18.,-2.20436423846524E-15,25.));
#10007=CARTESIAN_POINT('Origin',(-20.,-2.44929359829471E-15,25.));
#10008=CARTESIAN_POINT('',(-20.,-13.,23.));
#10009=CARTESIAN_POINT('',(-20.,-2.,23.));
#10010=CARTESIAN_POINT('',(-20.,-3.93203987888076E-15,23.));
#10011=CARTESIAN_POINT('',(-20.,-2.,2.));
#10012=CARTESIAN_POINT('',(-20.,-2.,25.));
#10013=CARTESIAN_POINT('',(-20.,-13.,2.));
#10014=CARTESIAN_POINT('',(-20.,-2.44929359829471E-15,2.));
#10015=CARTESIAN_POINT('',(-20.,-13.,25.));
#10016=CARTESIAN_POINT('Origin',(-20.,-15.,25.));
#10017=CARTESIAN_POINT('',(30.,-15.,23.));
#10018=CARTESIAN_POINT('',(-18.,-15.,23.));
#10019=CARTESIAN_POINT('',(-20.,-15.,23.));
#10020=CARTESIAN_POINT('',(-18.,-15.,2.));
#10021=CARTESIAN_POINT('',(-18.,-15.,25.));
#10022=CARTESIAN_POINT('',(30.,-15.,2.));
#10023=CARTESIAN_POINT('',(-20.,-15.,2.));
#10024=CARTESIAN_POINT('',(30.,-15.,25.));
#10025=CARTESIAN_POINT('Origin',(32.,86.8498045122456,25.));
#10026=CARTESIAN_POINT('',(32.,84.6000761633705,23.));
#10027=CARTESIAN_POINT('',(32.,-13.,23.));
#10028=CARTESIAN_POINT('',(32.,-15.,23.));
#10029=CARTESIAN_POINT('',(32.,-13.,2.));
#10030=CARTESIAN_POINT('',(32.,-13.,25.));
#10031=CARTESIAN_POINT('',(32.,86.8498045122456,2.));
#10032=CARTESIAN_POINT('',(32.,84.6000761633705,25.));
#10033=CARTESIAN_POINT('Origin',(-3.28761363381793,19.7279394918662,25.));
#10034=CARTESIAN_POINT('',(30.,84.6000761633705,25.));
#10035=CARTESIAN_POINT('',(1.74109754333981,78.4546297413593,25.));
#10036=CARTESIAN_POINT('Origin',(50.,-75.4117474694202,25.));
#10037=CARTESIAN_POINT('Origin',(55.3717972015101,68.8171894196414,25.));
#10038=CARTESIAN_POINT('',(-0.169896300137657,-2.,25.));
#10039=CARTESIAN_POINT('Origin',(-0.169896300137657,2.,25.));
#10040=CARTESIAN_POINT('',(-18.,-2.,25.));
#10041=CARTESIAN_POINT('',(-20.,-2.,25.));
#10042=CARTESIAN_POINT('',(-18.,-13.,25.));
#10043=CARTESIAN_POINT('',(-18.,-15.,25.));
#10044=CARTESIAN_POINT('',(30.,-13.,25.));
#10045=CARTESIAN_POINT('',(32.,-13.,25.));
#10046=CARTESIAN_POINT('',(30.,86.8498045122456,25.));
#10047=CARTESIAN_POINT('Origin',(-3.28761363381793,19.7279394918662,0.));
#10048=CARTESIAN_POINT('',(-0.169896300137657,-2.,0.));
#10049=CARTESIAN_POINT('Origin',(-0.169896300137657,2.,0.));
#10050=CARTESIAN_POINT('',(1.74109754333981,78.4546297413593,0.));
#10051=CARTESIAN_POINT('Origin',(55.3717972015101,68.8171894196414,0.));
#10052=CARTESIAN_POINT('Origin',(50.,-75.4117474694202,0.));
#10053=CARTESIAN_POINT('',(30.,-13.,0.));
#10054=CARTESIAN_POINT('',(30.,19.7279394918662,0.));
#10055=CARTESIAN_POINT('',(-18.,-13.,0.));
#10056=CARTESIAN_POINT('',(-3.28761363381793,-13.,0.));
#10057=CARTESIAN_POINT('',(-18.,-2.,0.));
#10058=CARTESIAN_POINT('',(-18.,19.7279394918662,0.));
#10059=CARTESIAN_POINT('',(-3.28761363381793,-2.,0.));
#10060=CARTESIAN_POINT('Origin',(23.,0.,7.5));
#10061=CARTESIAN_POINT('',(23.,93.3501340213216,7.5));
#10062=CARTESIAN_POINT('',(23.,0.,7.5));
#10063=CARTESIAN_POINT('',(23.,101.350134021322,15.5));
#10064=CARTESIAN_POINT('Origin',(23.,93.3501340213216,15.5));
#10065=CARTESIAN_POINT('',(23.,101.350134021322,7.5));
#10066=CARTESIAN_POINT('',(23.,90.0969828885913,22.5));
#10067=CARTESIAN_POINT('',(23.,90.0969828885913,22.5));
#10068=CARTESIAN_POINT('',(23.,85.5969828885913,22.5));
#10069=CARTESIAN_POINT('Origin',(8.00000000000006,2.19122965386546E-15,
7.5));
#10070=CARTESIAN_POINT('',(8.00000000000003,101.350134021322,15.5));
#10071=CARTESIAN_POINT('',(8.00000000000003,101.350134021322,7.5));
#10072=CARTESIAN_POINT('',(8.00000000000003,93.3501340213216,7.5));
#10073=CARTESIAN_POINT('Origin',(8.00000000000003,93.3501340213216,15.5));
#10074=CARTESIAN_POINT('',(8.00000000000006,2.19122965386546E-15,7.5));
#10075=CARTESIAN_POINT('',(8.00000000000004,90.0969828885913,22.5));
#10076=CARTESIAN_POINT('',(8.00000000000003,82.3501340213215,22.5));
#10077=CARTESIAN_POINT('',(8.00000000000004,90.0969828885913,22.5));
#10078=CARTESIAN_POINT('Origin',(0.,101.350134021322,7.5));
#10079=CARTESIAN_POINT('',(0.,101.350134021322,15.5));
#10080=CARTESIAN_POINT('Origin',(0.,0.,7.5));
#10081=CARTESIAN_POINT('',(0.,93.3501340213216,7.5));
#10082=CARTESIAN_POINT('Origin',(0.,93.3501340213216,15.5));
#10083=CARTESIAN_POINT('Origin',(8.00000000000004,90.0969828885913,22.5));
#10084=CARTESIAN_POINT('',(8.00000000000004,90.0969828885913,22.5));
#10085=CARTESIAN_POINT('Origin',(50.,-75.4117474694202,22.5));
#10086=CARTESIAN_POINT('Origin',(-20.,-13.,2.));
#10087=CARTESIAN_POINT('Origin',(-18.,-13.,2.));
#10088=CARTESIAN_POINT('Origin',(30.,-13.,2.));
#10089=CARTESIAN_POINT('Origin',(-18.,-13.,2.));
#10090=CARTESIAN_POINT('Origin',(-18.,-13.,2.));
#10091=CARTESIAN_POINT('Origin',(-18.,-13.,2.));
#10092=CARTESIAN_POINT('Origin',(30.,-13.,2.));
#10093=CARTESIAN_POINT('Origin',(30.,-13.,2.));
#10094=CARTESIAN_POINT('Origin',(30.,-13.,2.));
#10095=CARTESIAN_POINT('Origin',(-18.,-13.,25.));
#10096=CARTESIAN_POINT('Origin',(-18.,-13.,23.));
#10097=CARTESIAN_POINT('Origin',(-18.,-1.98670067136756E-15,2.));
#10098=CARTESIAN_POINT('Origin',(-18.,-2.,2.));
#10099=CARTESIAN_POINT('Origin',(30.,86.8498045122456,2.));
#10100=CARTESIAN_POINT('Origin',(30.,-13.,25.));
#10101=CARTESIAN_POINT('Origin',(30.,-13.,23.));
#10102=CARTESIAN_POINT('Origin',(-3.28761363381793,-13.,23.));
#10103=CARTESIAN_POINT('Origin',(-18.,-13.,23.));
#10104=CARTESIAN_POINT('Origin',(30.,-13.,23.));
#10105=CARTESIAN_POINT('Origin',(-18.,-13.,23.));
#10106=CARTESIAN_POINT('Origin',(-18.,-13.,23.));
#10107=CARTESIAN_POINT('Origin',(-18.,-2.,2.));
#10108=CARTESIAN_POINT('Origin',(-18.,-2.,2.));
#10109=CARTESIAN_POINT('Origin',(-18.,-2.,2.));
#10110=CARTESIAN_POINT('Origin',(30.,-13.,23.));
#10111=CARTESIAN_POINT('Origin',(30.,-13.,23.));
#10112=CARTESIAN_POINT('Origin',(-18.,19.7279394918662,23.));
#10113=CARTESIAN_POINT('Origin',(-18.,-2.,23.));
#10114=CARTESIAN_POINT('Origin',(-18.,-2.,25.));
#10115=CARTESIAN_POINT('Origin',(-18.,-2.,23.));
#10116=CARTESIAN_POINT('Origin',(2.44929359829471E-16,-2.,2.));
#10117=CARTESIAN_POINT('Origin',(-0.169896300137657,-2.,2.));
#10118=CARTESIAN_POINT('Origin',(55.3717972015101,68.8171894196414,2.));
#10119=CARTESIAN_POINT('Origin',(1.74109754333981,78.4546297413593,2.));
#10120=CARTESIAN_POINT('Origin',(50.,-75.4117474694202,2.));
#10121=CARTESIAN_POINT('Origin',(1.74109754333982,78.4546297413593,2.));
#10122=CARTESIAN_POINT('Origin',(30.,84.6000761633705,25.));
#10123=CARTESIAN_POINT('Origin',(30.,84.6000761633705,23.));
#10124=CARTESIAN_POINT('Origin',(30.,19.7279394918662,23.));
#10125=CARTESIAN_POINT('Origin',(30.,84.6000761633705,23.));
#10126=CARTESIAN_POINT('Origin',(-18.,-2.,23.));
#10127=CARTESIAN_POINT('Origin',(-18.,-2.,23.));
#10128=CARTESIAN_POINT('Origin',(-0.169896300137657,2.,2.));
#10129=CARTESIAN_POINT('Origin',(-0.169896300137657,2.,2.));
#10130=CARTESIAN_POINT('Origin',(1.74109754333981,78.4546297413593,2.));
#10131=CARTESIAN_POINT('Origin',(1.74109754333981,78.4546297413593,2.));
#10132=CARTESIAN_POINT('Origin',(30.,84.6000761633705,23.));
#10133=CARTESIAN_POINT('Origin',(30.,84.6000761633705,23.));
#10134=CARTESIAN_POINT('Origin',(-3.28761363381793,-2.,23.));
#10135=CARTESIAN_POINT('Origin',(-0.169896300137657,-2.,23.));
#10136=CARTESIAN_POINT('Origin',(-0.169896300137657,2.,25.));
#10137=CARTESIAN_POINT('Origin',(-0.169896300137657,2.,23.));
#10138=CARTESIAN_POINT('Origin',(1.74109754333982,78.4546297413593,25.));
#10139=CARTESIAN_POINT('Origin',(1.74109754333982,78.4546297413593,23.));
#10140=CARTESIAN_POINT('Origin',(50.,-75.4117474694202,23.));
#10141=CARTESIAN_POINT('Origin',(1.74109754333981,78.4546297413593,23.));
#10142=CARTESIAN_POINT('Origin',(-0.169896300137657,2.,23.));
#10143=CARTESIAN_POINT('Origin',(1.74109754333981,78.4546297413593,23.));
#10144=CARTESIAN_POINT('Origin',(1.74109754333981,78.4546297413593,23.));
#10145=CARTESIAN_POINT('Origin',(55.3717972015101,68.8171894196414,23.));
#10146=CARTESIAN_POINT('Origin',(-3.58124390253522,-5.29115334922921,5.70951949982205));
#10147=CARTESIAN_POINT('',(-5.15759532720172,-6.25691439705264,9.86573616141742));
#10148=CARTESIAN_POINT('',(-5.15759532720173,-4.03981623667055,1.63018293974891));
#10149=CARTESIAN_POINT('Origin',(-5.06582345881426,-6.27532846007085,9.90101997972383));
#10150=CARTESIAN_POINT('',(0.181310525678022,-7.32816804537255,11.918402053243));
#10151=CARTESIAN_POINT('Origin',(-0.0959656635925021,-4.00763402631843,
-0.315877705231196));
#10152=CARTESIAN_POINT('',(0.0234743673904921,-4.00687461789525,-0.361799188859744));
#10153=CARTESIAN_POINT('Origin',(11.453888025434,17.5975259767542,29.7255459071844));
#10154=CARTESIAN_POINT('Origin',(9.85030394827583,-2.21549538421888,-10.5620593400126));
#13149=UNCERTAINTY_MEASURE_WITH_UNIT(LENGTH_MEASURE(0.01),#13200,
'DISTANCE_ACCURACY_VALUE',
'Maximum model space distance between geometric entities at asserted c
onnectivities');
#13173=UNCERTAINTY_MEASURE_WITH_UNIT(LENGTH_MEASURE(0.01),#13200,
'DISTANCE_ACCURACY_VALUE',
'Maximum model space distance between geometric entities at asserted c
onnectivities');
#13175=(
GEOMETRIC_REPRESENTATION_CONTEXT(3)
GLOBAL_UNCERTAINTY_ASSIGNED_CONTEXT((#13149))
GLOBAL_UNIT_ASSIGNED_CONTEXT((#13200,#13202,#13203))
REPRESENTATION_CONTEXT('','3D')
);
#13199=(
GEOMETRIC_REPRESENTATION_CONTEXT(3)
GLOBAL_UNCERTAINTY_ASSIGNED_CONTEXT((#13173))
GLOBAL_UNIT_ASSIGNED_CONTEXT((#13200,#13202,#13203))
REPRESENTATION_CONTEXT('','3D')
);
#13200=(
LENGTH_UNIT()
NAMED_UNIT(*)
SI_UNIT(.MILLI.,.METRE.)
);
#13202=(
NAMED_UNIT(*)
PLANE_ANGLE_UNIT()
SI_UNIT($,.RADIAN.)
);
#13203=(
NAMED_UNIT(*)
SI_UNIT($,.STERADIAN.)
SOLID_ANGLE_UNIT()
);
#13205=SHAPE_DEFINITION_REPRESENTATION(#13230,#13279);
#13230=PRODUCT_DEFINITION_SHAPE('',$,#13305);
#13279=SHAPE_REPRESENTATION('',(#7061),#13175);
#13303=PRODUCT_DEFINITION_CONTEXT('part definition',#13380,'design');
#13305=PRODUCT_DEFINITION('Base','Base',#13330,#13303);
#13330=PRODUCT_DEFINITION_FORMATION('',$,#13383);
#13380=APPLICATION_CONTEXT(
'Core Data for Automotive Mechanical Design Process');
#13381=PRODUCT_CONTEXT('part definition',#13380,'mechanical');
#13383=PRODUCT('Base','Base','Base',(#13381));
#13408=PRESENTATION_STYLE_ASSIGNMENT((#13413));
#13413=SURFACE_STYLE_USAGE(.BOTH.,#13418);
#13418=SURFACE_SIDE_STYLE('',(#13423));
#13423=SURFACE_STYLE_FILL_AREA(#13428);
#13428=FILL_AREA_STYLE('Opaque(20,51,87)',(#13433));
#13433=FILL_AREA_STYLE_COLOUR('Opaque(20,51,87)',#13438);
#13438=COLOUR_RGB('Opaque(20,51,87)',0.0784313725490196,0.2,0.341176470588235);
ENDSEC;
END-ISO-10303-21;
